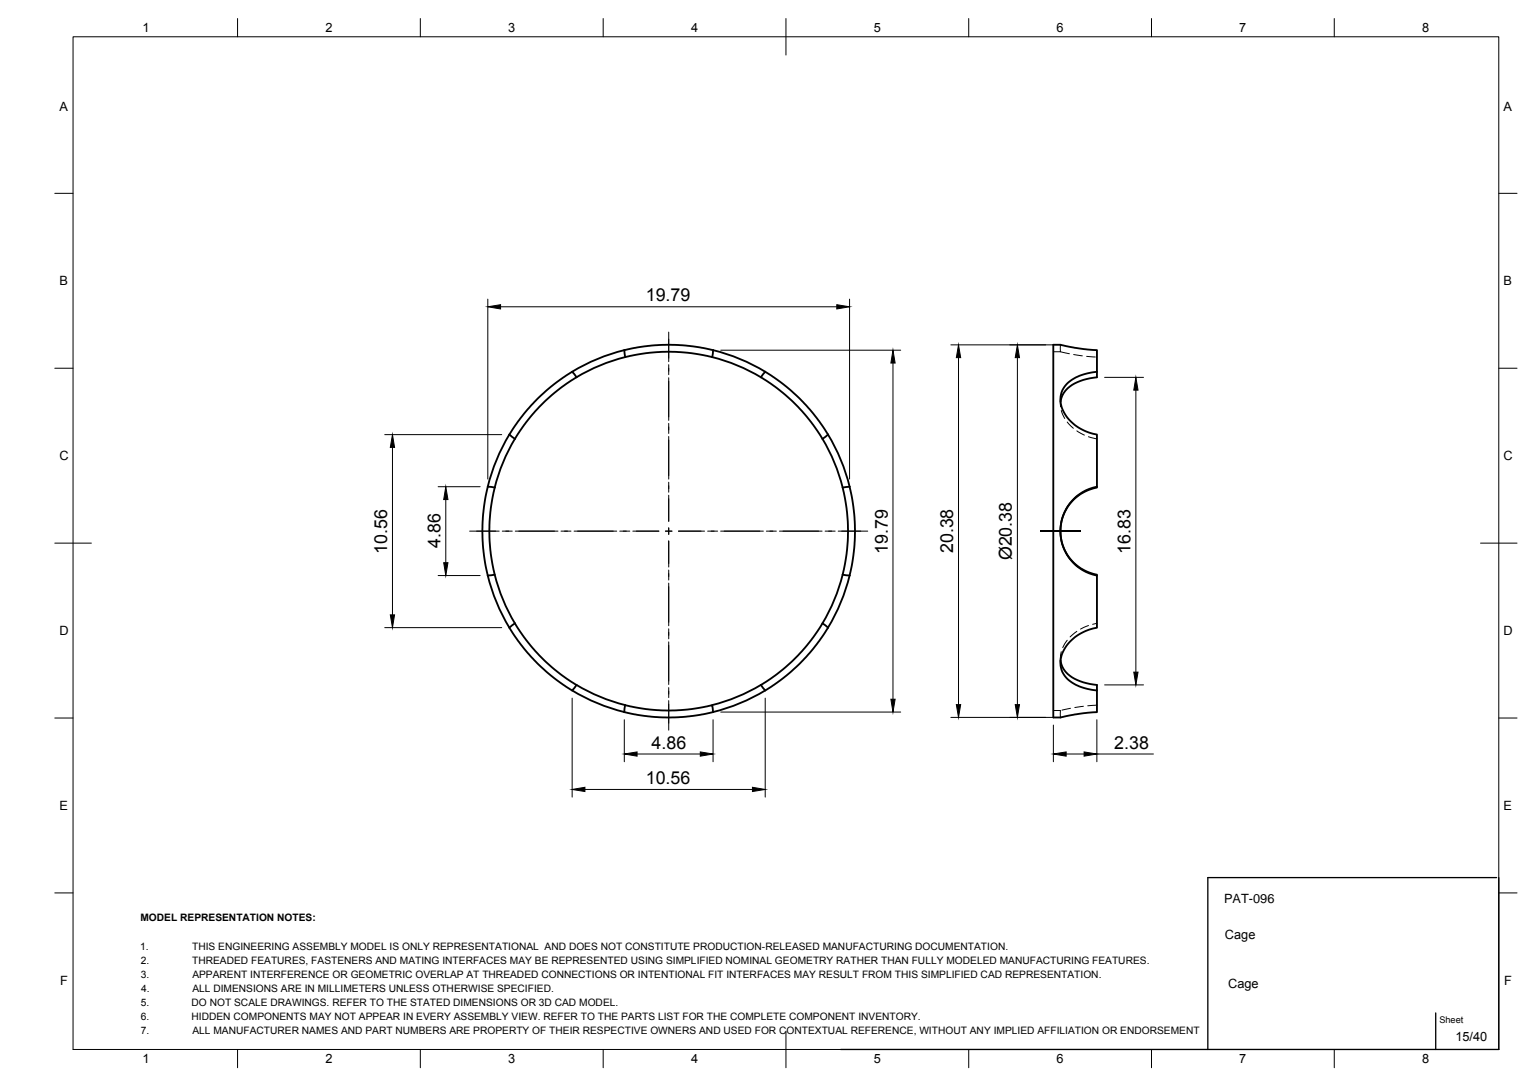
ISO-10303-21;
HEADER;
/* Generated by software containing ST-Developer
 * from STEP Tools, Inc. (www.steptools.com) 
 */

FILE_DESCRIPTION(
/* description */ ('PAT-096'),
/* implementation_level */ '2;1');

FILE_NAME(
/* name */ 'Cage.step',
/* time_stamp */ '2026-10-29T17:03:14-07:00',
/* author */ (''),
/* organization */ (''),
/* preprocessor_version */ 'ST-DEVELOPER v20.2',
/* originating_system */ 'Autodesk Translation Framework v15.17.0.0',
/* authorisation */ '');

FILE_SCHEMA (('AUTOMOTIVE_DESIGN { 1 0 10303 214 3 1 1 }'));
ENDSEC;

DATA;
#10=MECHANICAL_DESIGN_GEOMETRIC_PRESENTATION_REPRESENTATION('',(#412),#10650);
#271=SPHERICAL_SURFACE('',#6142,0.247676);
#272=SPHERICAL_SURFACE('',#6158,0.247676);
#273=SPHERICAL_SURFACE('',#6163,0.247676);
#274=SPHERICAL_SURFACE('',#6168,0.247676);
#275=SPHERICAL_SURFACE('',#6173,0.247676);
#276=SPHERICAL_SURFACE('',#6178,0.247676);
#277=SPHERICAL_SURFACE('',#6183,0.247676);
#278=SPHERICAL_SURFACE('',#6191,0.247676);
#285=B_SPLINE_CURVE_WITH_KNOTS('',3,(#9044,#9045,#9046,#9047,#9048,#9049,
#9050,#9051,#9052,#9053,#9054,#9055,#9056,#9057,#9058,#9059,#9060,#9061,
#9062,#9063,#9064,#9065),.UNSPECIFIED.,.F.,.F.,(4,2,2,2,2,2,2,2,2,2,4),
(0.0473477652366656,0.126350602536658,0.189525903804987,0.252701205073317,
0.313298422430275,0.373895639787233,0.434492857144191,0.495090074501149,
0.558265375769478,0.621440677037807,0.7004435143378),.UNSPECIFIED.);
#286=B_SPLINE_CURVE_WITH_KNOTS('',3,(#9069,#9070,#9071,#9072,#9073,#9074,
#9075,#9076,#9077,#9078,#9079,#9080,#9081,#9082,#9083,#9084,#9085,#9086,
#9087,#9088,#9089,#9090),.UNSPECIFIED.,.F.,.F.,(4,2,2,2,2,2,2,2,2,2,4),
(0.0464897534940957,0.0852567806515119,0.170513561303024,0.246687263103517,
0.308657850341199,0.370628437578881,0.432599024816563,0.494569612054245,
0.570743313854739,0.656000094506251,0.694767121663666),.UNSPECIFIED.);
#287=B_SPLINE_CURVE_WITH_KNOTS('',3,(#9096,#9097,#9098,#9099,#9100,#9101,
#9102,#9103,#9104,#9105,#9106,#9107,#9108,#9109,#9110,#9111,#9112,#9113,
#9114,#9115,#9116,#9117),.UNSPECIFIED.,.F.,.F.,(4,2,2,2,2,2,2,2,2,2,4),
(0.0464897534940957,0.0852567806515118,0.170513561303024,0.246687263103517,
0.308657850341199,0.370628437578881,0.432599024816563,0.494569612054245,
0.570743313854738,0.65600009450625,0.694767121663666),.UNSPECIFIED.);
#288=B_SPLINE_CURVE_WITH_KNOTS('',3,(#9121,#9122,#9123,#9124,#9125,#9126,
#9127,#9128,#9129,#9130,#9131,#9132,#9133,#9134,#9135,#9136,#9137,#9138,
#9139,#9140,#9141,#9142),.UNSPECIFIED.,.F.,.F.,(4,2,2,2,2,2,2,2,2,2,4),
(0.0464897534940957,0.0852567806515119,0.170513561303024,0.246687263103517,
0.308657850341199,0.370628437578881,0.432599024816563,0.494569612054245,
0.570743313854739,0.656000094506251,0.694767121663666),.UNSPECIFIED.);
#289=B_SPLINE_CURVE_WITH_KNOTS('',3,(#9146,#9147,#9148,#9149,#9150,#9151,
#9152,#9153,#9154,#9155,#9156,#9157),.UNSPECIFIED.,.F.,.F.,(4,2,2,2,2,4),
(0.0464897534940957,0.0852567806515119,0.170513561303024,0.246687263103517,
0.308657850341199,0.370628437578881),.UNSPECIFIED.);
#290=B_SPLINE_CURVE_WITH_KNOTS('',3,(#9162,#9163,#9164,#9165,#9166,#9167,
#9168,#9169,#9170,#9171,#9172,#9173),.UNSPECIFIED.,.F.,.F.,(4,2,2,2,2,4),
(0.370628437578881,0.432599024816563,0.494569612054245,0.570743313854738,
0.65600009450625,0.694767121663666),.UNSPECIFIED.);
#291=B_SPLINE_CURVE_WITH_KNOTS('',3,(#9177,#9178,#9179,#9180,#9181,#9182,
#9183,#9184,#9185,#9186,#9187,#9188,#9189,#9190,#9191,#9192,#9193,#9194,
#9195,#9196,#9197,#9198),.UNSPECIFIED.,.F.,.F.,(4,2,2,2,2,2,2,2,2,2,4),
(0.0464897534940957,0.0852567806515121,0.170513561303024,0.246687263103518,
0.308657850341199,0.370628437578881,0.432599024816563,0.494569612054245,
0.570743313854738,0.65600009450625,0.694767121663666),.UNSPECIFIED.);
#292=B_SPLINE_CURVE_WITH_KNOTS('',3,(#9202,#9203,#9204,#9205,#9206,#9207,
#9208,#9209,#9210,#9211,#9212,#9213,#9214,#9215,#9216,#9217,#9218,#9219,
#9220,#9221,#9222,#9223),.UNSPECIFIED.,.F.,.F.,(4,2,2,2,2,2,2,2,2,2,4),
(0.0464897534940957,0.0852567806515119,0.170513561303024,0.246687263103517,
0.308657850341199,0.370628437578881,0.432599024816563,0.494569612054245,
0.570743313854738,0.65600009450625,0.694767121663667),.UNSPECIFIED.);
#293=B_SPLINE_CURVE_WITH_KNOTS('',3,(#9227,#9228,#9229,#9230,#9231,#9232,
#9233,#9234,#9235,#9236,#9237,#9238,#9239,#9240,#9241,#9242,#9243,#9244,
#9245,#9246,#9247,#9248),.UNSPECIFIED.,.F.,.F.,(4,2,2,2,2,2,2,2,2,2,4),
(0.0464897534940957,0.0852567806515119,0.170513561303024,0.246687263103517,
0.308657850341199,0.370628437578881,0.432599024816563,0.494569612054245,
0.570743313854738,0.65600009450625,0.694767121663666),.UNSPECIFIED.);
#294=B_SPLINE_CURVE_WITH_KNOTS('',3,(#9252,#9253,#9254,#9255,#9256,#9257,
#9258,#9259,#9260,#9261,#9262,#9263,#9264,#9265,#9266,#9267,#9268,#9269,
#9270,#9271,#9272,#9273),.UNSPECIFIED.,.F.,.F.,(4,2,2,2,2,2,2,2,2,2,4),
(0.0464897534940957,0.0852567806515119,0.170513561303024,0.246687263103517,
0.308657850341199,0.370628437578881,0.432599024816563,0.494569612054245,
0.570743313854739,0.656000094506251,0.694767121663667),.UNSPECIFIED.);
#295=B_SPLINE_CURVE_WITH_KNOTS('',3,(#9281,#9282,#9283,#9284,#9285,#9286,
#9287,#9288,#9289,#9290,#9291,#9292,#9293,#9294,#9295,#9296,#9297,#9298,
#9299,#9300,#9301,#9302),.UNSPECIFIED.,.F.,.F.,(4,2,2,2,2,2,2,2,2,2,4),
(0.0473477652366656,0.126350602536658,0.189525903804987,0.252701205073316,
0.313298422430274,0.373895639787232,0.434492857144191,0.495090074501149,
0.558265375769478,0.621440677037807,0.7004435143378),.UNSPECIFIED.);
#296=B_SPLINE_CURVE_WITH_KNOTS('',3,(#9310,#9311,#9312,#9313,#9314,#9315,
#9316,#9317,#9318,#9319,#9320,#9321,#9322,#9323,#9324,#9325,#9326,#9327,
#9328,#9329,#9330,#9331),.UNSPECIFIED.,.F.,.F.,(4,2,2,2,2,2,2,2,2,2,4),
(0.0473477652366656,0.126350602536658,0.189525903804987,0.252701205073317,
0.313298422430275,0.373895639787233,0.434492857144191,0.495090074501149,
0.558265375769478,0.621440677037807,0.7004435143378),.UNSPECIFIED.);
#297=B_SPLINE_CURVE_WITH_KNOTS('',3,(#9340,#9341,#9342,#9343,#9344,#9345,
#9346,#9347,#9348,#9349,#9350,#9351),.UNSPECIFIED.,.F.,.F.,(4,2,2,2,2,4),
(0.0473477652366656,0.126350602536658,0.189525903804987,0.252701205073316,
0.313298422430275,0.373895639787233),.UNSPECIFIED.);
#298=B_SPLINE_CURVE_WITH_KNOTS('',3,(#9353,#9354,#9355,#9356,#9357,#9358,
#9359,#9360,#9361,#9362,#9363,#9364),.UNSPECIFIED.,.F.,.F.,(4,2,2,2,2,4),
(0.373895639787233,0.434492857144191,0.495090074501149,0.558265375769478,
0.621440677037807,0.7004435143378),.UNSPECIFIED.);
#299=B_SPLINE_CURVE_WITH_KNOTS('',3,(#9371,#9372,#9373,#9374,#9375,#9376,
#9377,#9378,#9379,#9380,#9381,#9382,#9383,#9384,#9385,#9386,#9387,#9388,
#9389,#9390,#9391,#9392),.UNSPECIFIED.,.F.,.F.,(4,2,2,2,2,2,2,2,2,2,4),
(0.0473477652366656,0.126350602536658,0.189525903804987,0.252701205073316,
0.313298422430275,0.373895639787233,0.434492857144191,0.495090074501149,
0.558265375769478,0.621440677037807,0.7004435143378),.UNSPECIFIED.);
#300=B_SPLINE_CURVE_WITH_KNOTS('',3,(#9400,#9401,#9402,#9403,#9404,#9405,
#9406,#9407,#9408,#9409,#9410,#9411,#9412,#9413,#9414,#9415,#9416,#9417,
#9418,#9419,#9420,#9421),.UNSPECIFIED.,.F.,.F.,(4,2,2,2,2,2,2,2,2,2,4),
(0.0473477652366656,0.126350602536658,0.189525903804987,0.252701205073317,
0.313298422430275,0.373895639787233,0.434492857144191,0.495090074501149,
0.558265375769478,0.621440677037807,0.7004435143378),.UNSPECIFIED.);
#301=B_SPLINE_CURVE_WITH_KNOTS('',3,(#9429,#9430,#9431,#9432,#9433,#9434,
#9435,#9436,#9437,#9438,#9439,#9440,#9441,#9442,#9443,#9444,#9445,#9446,
#9447,#9448,#9449,#9450),.UNSPECIFIED.,.F.,.F.,(4,2,2,2,2,2,2,2,2,2,4),
(0.0473477652366656,0.126350602536658,0.189525903804987,0.252701205073316,
0.313298422430275,0.373895639787233,0.434492857144191,0.495090074501149,
0.558265375769478,0.621440677037807,0.7004435143378),.UNSPECIFIED.);
#302=B_SPLINE_CURVE_WITH_KNOTS('',3,(#9459,#9460,#9461,#9462,#9463,#9464,
#9465,#9466,#9467,#9468,#9469,#9470,#9471,#9472,#9473,#9474,#9475,#9476,
#9477,#9478,#9479,#9480),.UNSPECIFIED.,.F.,.F.,(4,2,2,2,2,2,2,2,2,2,4),
(0.0473477652366656,0.126350602536658,0.189525903804987,0.252701205073317,
0.313298422430275,0.373895639787233,0.434492857144191,0.495090074501149,
0.558265375769478,0.621440677037807,0.7004435143378),.UNSPECIFIED.);
#343=SHAPE_REPRESENTATION_RELATIONSHIP('SRR','None',#10804,#374);
#374=ADVANCED_BREP_SHAPE_REPRESENTATION('',(#450),#10622);
#412=STYLED_ITEM('',(#11064),#450);
#450=MANIFOLD_SOLID_BREP('Continuous crown cage',#5546);
#527=FACE_BOUND('',#1299,.T.);
#652=PLANE('',#6155);
#653=PLANE('',#6160);
#654=PLANE('',#6165);
#655=PLANE('',#6170);
#656=PLANE('',#6175);
#657=PLANE('',#6180);
#658=PLANE('',#6189);
#659=PLANE('',#6193);
#660=PLANE('',#6194);
#891=FACE_OUTER_BOUND('',#1281,.T.);
#892=FACE_OUTER_BOUND('',#1282,.T.);
#893=FACE_OUTER_BOUND('',#1283,.T.);
#894=FACE_OUTER_BOUND('',#1284,.T.);
#895=FACE_OUTER_BOUND('',#1285,.T.);
#896=FACE_OUTER_BOUND('',#1286,.T.);
#897=FACE_OUTER_BOUND('',#1287,.T.);
#898=FACE_OUTER_BOUND('',#1288,.T.);
#899=FACE_OUTER_BOUND('',#1289,.T.);
#900=FACE_OUTER_BOUND('',#1290,.T.);
#901=FACE_OUTER_BOUND('',#1291,.T.);
#902=FACE_OUTER_BOUND('',#1292,.T.);
#903=FACE_OUTER_BOUND('',#1293,.T.);
#904=FACE_OUTER_BOUND('',#1294,.T.);
#905=FACE_OUTER_BOUND('',#1295,.T.);
#906=FACE_OUTER_BOUND('',#1296,.T.);
#907=FACE_OUTER_BOUND('',#1297,.T.);
#908=FACE_OUTER_BOUND('',#1298,.T.);
#909=FACE_OUTER_BOUND('',#1300,.T.);
#1281=EDGE_LOOP('',(#4123,#4124,#4125,#4126));
#1282=EDGE_LOOP('',(#4127,#4128,#4129,#4130,#4131,#4132,#4133,#4134,#4135,
#4136,#4137,#4138,#4139,#4140,#4141,#4142,#4143,#4144,#4145,#4146));
#1283=EDGE_LOOP('',(#4147,#4148,#4149,#4150));
#1284=EDGE_LOOP('',(#4151,#4152,#4153,#4154));
#1285=EDGE_LOOP('',(#4155,#4156,#4157,#4158));
#1286=EDGE_LOOP('',(#4159,#4160,#4161,#4162));
#1287=EDGE_LOOP('',(#4163,#4164,#4165,#4166));
#1288=EDGE_LOOP('',(#4167,#4168,#4169,#4170,#4171,#4172));
#1289=EDGE_LOOP('',(#4173,#4174,#4175,#4176));
#1290=EDGE_LOOP('',(#4177,#4178,#4179,#4180));
#1291=EDGE_LOOP('',(#4181,#4182,#4183,#4184));
#1292=EDGE_LOOP('',(#4185,#4186,#4187,#4188));
#1293=EDGE_LOOP('',(#4189,#4190,#4191,#4192));
#1294=EDGE_LOOP('',(#4193,#4194,#4195,#4196));
#1295=EDGE_LOOP('',(#4197,#4198,#4199,#4200,#4201,#4202,#4203,#4204,#4205,
#4206,#4207,#4208,#4209,#4210,#4211,#4212,#4213,#4214,#4215,#4216));
#1296=EDGE_LOOP('',(#4217,#4218,#4219,#4220));
#1297=EDGE_LOOP('',(#4221,#4222,#4223,#4224));
#1298=EDGE_LOOP('',(#4225));
#1299=EDGE_LOOP('',(#4226));
#1300=EDGE_LOOP('',(#4227,#4228,#4229,#4230));
#1686=LINE('',#9159,#2015);
#1687=LINE('',#9455,#2016);
#2015=VECTOR('',#7224,1.019052);
#2016=VECTOR('',#7301,0.980948);
#2374=CIRCLE('',#6143,0.243053047864041);
#2375=CIRCLE('',#6144,0.243053047864041);
#2376=CIRCLE('',#6146,1.019052);
#2377=CIRCLE('',#6147,1.019052);
#2378=CIRCLE('',#6148,1.019052);
#2379=CIRCLE('',#6149,1.019052);
#2380=CIRCLE('',#6150,1.019052);
#2381=CIRCLE('',#6151,1.019052);
#2382=CIRCLE('',#6152,1.019052);
#2383=CIRCLE('',#6153,1.019052);
#2384=CIRCLE('',#6154,1.019052);
#2385=CIRCLE('',#6156,0.980948);
#2386=CIRCLE('',#6157,0.243053047864041);
#2387=CIRCLE('',#6159,0.243053047864041);
#2388=CIRCLE('',#6161,0.980948);
#2389=CIRCLE('',#6162,0.243053047864041);
#2390=CIRCLE('',#6164,0.243053047864041);
#2391=CIRCLE('',#6166,0.980948);
#2392=CIRCLE('',#6167,0.243053047864041);
#2393=CIRCLE('',#6169,0.243053047864041);
#2394=CIRCLE('',#6171,0.980948);
#2395=CIRCLE('',#6172,0.243053047864041);
#2396=CIRCLE('',#6174,0.243053047864041);
#2397=CIRCLE('',#6176,0.980948);
#2398=CIRCLE('',#6177,0.243053047864041);
#2399=CIRCLE('',#6179,0.243053047864041);
#2400=CIRCLE('',#6181,0.980948);
#2401=CIRCLE('',#6182,0.243053047864041);
#2402=CIRCLE('',#6184,0.243053047864041);
#2403=CIRCLE('',#6186,0.980948);
#2404=CIRCLE('',#6187,0.980948);
#2405=CIRCLE('',#6188,0.980948);
#2406=CIRCLE('',#6190,0.243053047864041);
#2407=CIRCLE('',#6192,0.243053047864041);
#2723=VERTEX_POINT('',#9042);
#2724=VERTEX_POINT('',#9043);
#2725=VERTEX_POINT('',#9066);
#2726=VERTEX_POINT('',#9068);
#2727=VERTEX_POINT('',#9093);
#2728=VERTEX_POINT('',#9095);
#2729=VERTEX_POINT('',#9118);
#2730=VERTEX_POINT('',#9120);
#2731=VERTEX_POINT('',#9143);
#2732=VERTEX_POINT('',#9145);
#2733=VERTEX_POINT('',#9158);
#2734=VERTEX_POINT('',#9161);
#2735=VERTEX_POINT('',#9174);
#2736=VERTEX_POINT('',#9176);
#2737=VERTEX_POINT('',#9199);
#2738=VERTEX_POINT('',#9201);
#2739=VERTEX_POINT('',#9224);
#2740=VERTEX_POINT('',#9226);
#2741=VERTEX_POINT('',#9249);
#2742=VERTEX_POINT('',#9251);
#2743=VERTEX_POINT('',#9276);
#2744=VERTEX_POINT('',#9280);
#2745=VERTEX_POINT('',#9305);
#2746=VERTEX_POINT('',#9309);
#2747=VERTEX_POINT('',#9334);
#2748=VERTEX_POINT('',#9338);
#2749=VERTEX_POINT('',#9339);
#2750=VERTEX_POINT('',#9366);
#2751=VERTEX_POINT('',#9370);
#2752=VERTEX_POINT('',#9395);
#2753=VERTEX_POINT('',#9399);
#2754=VERTEX_POINT('',#9424);
#2755=VERTEX_POINT('',#9428);
#2756=VERTEX_POINT('',#9453);
#2757=VERTEX_POINT('',#9456);
#2758=VERTEX_POINT('',#9458);
#3240=EDGE_CURVE('',#2723,#2724,#285,.T.);
#3241=EDGE_CURVE('',#2725,#2723,#2374,.T.);
#3242=EDGE_CURVE('',#2726,#2725,#286,.T.);
#3243=EDGE_CURVE('',#2724,#2726,#2375,.T.);
#3244=EDGE_CURVE('',#2727,#2725,#2376,.T.);
#3245=EDGE_CURVE('',#2727,#2728,#287,.T.);
#3246=EDGE_CURVE('',#2729,#2728,#2377,.T.);
#3247=EDGE_CURVE('',#2729,#2730,#288,.T.);
#3248=EDGE_CURVE('',#2731,#2730,#2378,.T.);
#3249=EDGE_CURVE('',#2731,#2732,#289,.T.);
#3250=EDGE_CURVE('',#2732,#2733,#1686,.T.);
#3251=EDGE_CURVE('',#2733,#2733,#2379,.T.);
#3252=EDGE_CURVE('',#2732,#2734,#290,.T.);
#3253=EDGE_CURVE('',#2735,#2734,#2380,.T.);
#3254=EDGE_CURVE('',#2735,#2736,#291,.T.);
#3255=EDGE_CURVE('',#2737,#2736,#2381,.T.);
#3256=EDGE_CURVE('',#2737,#2738,#292,.T.);
#3257=EDGE_CURVE('',#2739,#2738,#2382,.T.);
#3258=EDGE_CURVE('',#2739,#2740,#293,.T.);
#3259=EDGE_CURVE('',#2741,#2740,#2383,.T.);
#3260=EDGE_CURVE('',#2741,#2742,#294,.T.);
#3261=EDGE_CURVE('',#2726,#2742,#2384,.T.);
#3262=EDGE_CURVE('',#2723,#2743,#2385,.T.);
#3263=EDGE_CURVE('',#2743,#2727,#2386,.T.);
#3264=EDGE_CURVE('',#2744,#2743,#295,.T.);
#3265=EDGE_CURVE('',#2728,#2744,#2387,.T.);
#3266=EDGE_CURVE('',#2744,#2745,#2388,.T.);
#3267=EDGE_CURVE('',#2745,#2729,#2389,.T.);
#3268=EDGE_CURVE('',#2746,#2745,#296,.T.);
#3269=EDGE_CURVE('',#2730,#2746,#2390,.T.);
#3270=EDGE_CURVE('',#2746,#2747,#2391,.T.);
#3271=EDGE_CURVE('',#2747,#2731,#2392,.T.);
#3272=EDGE_CURVE('',#2748,#2749,#297,.T.);
#3273=EDGE_CURVE('',#2734,#2748,#2393,.T.);
#3274=EDGE_CURVE('',#2749,#2747,#298,.T.);
#3275=EDGE_CURVE('',#2748,#2750,#2394,.T.);
#3276=EDGE_CURVE('',#2750,#2735,#2395,.T.);
#3277=EDGE_CURVE('',#2751,#2750,#299,.T.);
#3278=EDGE_CURVE('',#2736,#2751,#2396,.T.);
#3279=EDGE_CURVE('',#2751,#2752,#2397,.T.);
#3280=EDGE_CURVE('',#2752,#2737,#2398,.T.);
#3281=EDGE_CURVE('',#2753,#2752,#300,.T.);
#3282=EDGE_CURVE('',#2738,#2753,#2399,.T.);
#3283=EDGE_CURVE('',#2753,#2754,#2400,.T.);
#3284=EDGE_CURVE('',#2754,#2739,#2401,.T.);
#3285=EDGE_CURVE('',#2755,#2754,#301,.T.);
#3286=EDGE_CURVE('',#2740,#2755,#2402,.T.);
#3287=EDGE_CURVE('',#2756,#2756,#2403,.T.);
#3288=EDGE_CURVE('',#2756,#2749,#1687,.T.);
#3289=EDGE_CURVE('',#2757,#2724,#2404,.T.);
#3290=EDGE_CURVE('',#2757,#2758,#302,.T.);
#3291=EDGE_CURVE('',#2755,#2758,#2405,.T.);
#3292=EDGE_CURVE('',#2742,#2757,#2406,.T.);
#3293=EDGE_CURVE('',#2758,#2741,#2407,.T.);
#4123=ORIENTED_EDGE('',*,*,#3240,.F.);
#4124=ORIENTED_EDGE('',*,*,#3241,.F.);
#4125=ORIENTED_EDGE('',*,*,#3242,.F.);
#4126=ORIENTED_EDGE('',*,*,#3243,.F.);
#4127=ORIENTED_EDGE('',*,*,#3242,.T.);
#4128=ORIENTED_EDGE('',*,*,#3244,.F.);
#4129=ORIENTED_EDGE('',*,*,#3245,.T.);
#4130=ORIENTED_EDGE('',*,*,#3246,.F.);
#4131=ORIENTED_EDGE('',*,*,#3247,.T.);
#4132=ORIENTED_EDGE('',*,*,#3248,.F.);
#4133=ORIENTED_EDGE('',*,*,#3249,.T.);
#4134=ORIENTED_EDGE('',*,*,#3250,.T.);
#4135=ORIENTED_EDGE('',*,*,#3251,.F.);
#4136=ORIENTED_EDGE('',*,*,#3250,.F.);
#4137=ORIENTED_EDGE('',*,*,#3252,.T.);
#4138=ORIENTED_EDGE('',*,*,#3253,.F.);
#4139=ORIENTED_EDGE('',*,*,#3254,.T.);
#4140=ORIENTED_EDGE('',*,*,#3255,.F.);
#4141=ORIENTED_EDGE('',*,*,#3256,.T.);
#4142=ORIENTED_EDGE('',*,*,#3257,.F.);
#4143=ORIENTED_EDGE('',*,*,#3258,.T.);
#4144=ORIENTED_EDGE('',*,*,#3259,.F.);
#4145=ORIENTED_EDGE('',*,*,#3260,.T.);
#4146=ORIENTED_EDGE('',*,*,#3261,.F.);
#4147=ORIENTED_EDGE('',*,*,#3241,.T.);
#4148=ORIENTED_EDGE('',*,*,#3262,.T.);
#4149=ORIENTED_EDGE('',*,*,#3263,.T.);
#4150=ORIENTED_EDGE('',*,*,#3244,.T.);
#4151=ORIENTED_EDGE('',*,*,#3264,.F.);
#4152=ORIENTED_EDGE('',*,*,#3265,.F.);
#4153=ORIENTED_EDGE('',*,*,#3245,.F.);
#4154=ORIENTED_EDGE('',*,*,#3263,.F.);
#4155=ORIENTED_EDGE('',*,*,#3265,.T.);
#4156=ORIENTED_EDGE('',*,*,#3266,.T.);
#4157=ORIENTED_EDGE('',*,*,#3267,.T.);
#4158=ORIENTED_EDGE('',*,*,#3246,.T.);
#4159=ORIENTED_EDGE('',*,*,#3268,.F.);
#4160=ORIENTED_EDGE('',*,*,#3269,.F.);
#4161=ORIENTED_EDGE('',*,*,#3247,.F.);
#4162=ORIENTED_EDGE('',*,*,#3267,.F.);
#4163=ORIENTED_EDGE('',*,*,#3269,.T.);
#4164=ORIENTED_EDGE('',*,*,#3270,.T.);
#4165=ORIENTED_EDGE('',*,*,#3271,.T.);
#4166=ORIENTED_EDGE('',*,*,#3248,.T.);
#4167=ORIENTED_EDGE('',*,*,#3272,.F.);
#4168=ORIENTED_EDGE('',*,*,#3273,.F.);
#4169=ORIENTED_EDGE('',*,*,#3252,.F.);
#4170=ORIENTED_EDGE('',*,*,#3249,.F.);
#4171=ORIENTED_EDGE('',*,*,#3271,.F.);
#4172=ORIENTED_EDGE('',*,*,#3274,.F.);
#4173=ORIENTED_EDGE('',*,*,#3273,.T.);
#4174=ORIENTED_EDGE('',*,*,#3275,.T.);
#4175=ORIENTED_EDGE('',*,*,#3276,.T.);
#4176=ORIENTED_EDGE('',*,*,#3253,.T.);
#4177=ORIENTED_EDGE('',*,*,#3277,.F.);
#4178=ORIENTED_EDGE('',*,*,#3278,.F.);
#4179=ORIENTED_EDGE('',*,*,#3254,.F.);
#4180=ORIENTED_EDGE('',*,*,#3276,.F.);
#4181=ORIENTED_EDGE('',*,*,#3278,.T.);
#4182=ORIENTED_EDGE('',*,*,#3279,.T.);
#4183=ORIENTED_EDGE('',*,*,#3280,.T.);
#4184=ORIENTED_EDGE('',*,*,#3255,.T.);
#4185=ORIENTED_EDGE('',*,*,#3281,.F.);
#4186=ORIENTED_EDGE('',*,*,#3282,.F.);
#4187=ORIENTED_EDGE('',*,*,#3256,.F.);
#4188=ORIENTED_EDGE('',*,*,#3280,.F.);
#4189=ORIENTED_EDGE('',*,*,#3282,.T.);
#4190=ORIENTED_EDGE('',*,*,#3283,.T.);
#4191=ORIENTED_EDGE('',*,*,#3284,.T.);
#4192=ORIENTED_EDGE('',*,*,#3257,.T.);
#4193=ORIENTED_EDGE('',*,*,#3258,.F.);
#4194=ORIENTED_EDGE('',*,*,#3284,.F.);
#4195=ORIENTED_EDGE('',*,*,#3285,.F.);
#4196=ORIENTED_EDGE('',*,*,#3286,.F.);
#4197=ORIENTED_EDGE('',*,*,#3287,.F.);
#4198=ORIENTED_EDGE('',*,*,#3288,.T.);
#4199=ORIENTED_EDGE('',*,*,#3274,.T.);
#4200=ORIENTED_EDGE('',*,*,#3270,.F.);
#4201=ORIENTED_EDGE('',*,*,#3268,.T.);
#4202=ORIENTED_EDGE('',*,*,#3266,.F.);
#4203=ORIENTED_EDGE('',*,*,#3264,.T.);
#4204=ORIENTED_EDGE('',*,*,#3262,.F.);
#4205=ORIENTED_EDGE('',*,*,#3240,.T.);
#4206=ORIENTED_EDGE('',*,*,#3289,.F.);
#4207=ORIENTED_EDGE('',*,*,#3290,.T.);
#4208=ORIENTED_EDGE('',*,*,#3291,.F.);
#4209=ORIENTED_EDGE('',*,*,#3285,.T.);
#4210=ORIENTED_EDGE('',*,*,#3283,.F.);
#4211=ORIENTED_EDGE('',*,*,#3281,.T.);
#4212=ORIENTED_EDGE('',*,*,#3279,.F.);
#4213=ORIENTED_EDGE('',*,*,#3277,.T.);
#4214=ORIENTED_EDGE('',*,*,#3275,.F.);
#4215=ORIENTED_EDGE('',*,*,#3272,.T.);
#4216=ORIENTED_EDGE('',*,*,#3288,.F.);
#4217=ORIENTED_EDGE('',*,*,#3243,.T.);
#4218=ORIENTED_EDGE('',*,*,#3261,.T.);
#4219=ORIENTED_EDGE('',*,*,#3292,.T.);
#4220=ORIENTED_EDGE('',*,*,#3289,.T.);
#4221=ORIENTED_EDGE('',*,*,#3260,.F.);
#4222=ORIENTED_EDGE('',*,*,#3293,.F.);
#4223=ORIENTED_EDGE('',*,*,#3290,.F.);
#4224=ORIENTED_EDGE('',*,*,#3292,.F.);
#4225=ORIENTED_EDGE('',*,*,#3251,.T.);
#4226=ORIENTED_EDGE('',*,*,#3287,.T.);
#4227=ORIENTED_EDGE('',*,*,#3286,.T.);
#4228=ORIENTED_EDGE('',*,*,#3291,.T.);
#4229=ORIENTED_EDGE('',*,*,#3293,.T.);
#4230=ORIENTED_EDGE('',*,*,#3259,.T.);
#5117=CYLINDRICAL_SURFACE('',#6145,1.019052);
#5118=CYLINDRICAL_SURFACE('',#6185,0.980948);
#5296=ADVANCED_FACE('',(#891),#271,.F.);
#5297=ADVANCED_FACE('',(#892),#5117,.T.);
#5298=ADVANCED_FACE('',(#893),#652,.T.);
#5299=ADVANCED_FACE('',(#894),#272,.F.);
#5300=ADVANCED_FACE('',(#895),#653,.T.);
#5301=ADVANCED_FACE('',(#896),#273,.F.);
#5302=ADVANCED_FACE('',(#897),#654,.T.);
#5303=ADVANCED_FACE('',(#898),#274,.F.);
#5304=ADVANCED_FACE('',(#899),#655,.T.);
#5305=ADVANCED_FACE('',(#900),#275,.F.);
#5306=ADVANCED_FACE('',(#901),#656,.T.);
#5307=ADVANCED_FACE('',(#902),#276,.F.);
#5308=ADVANCED_FACE('',(#903),#657,.T.);
#5309=ADVANCED_FACE('',(#904),#277,.F.);
#5310=ADVANCED_FACE('',(#905),#5118,.F.);
#5311=ADVANCED_FACE('',(#906),#658,.T.);
#5312=ADVANCED_FACE('',(#907),#278,.F.);
#5313=ADVANCED_FACE('',(#908,#527),#659,.T.);
#5314=ADVANCED_FACE('',(#909),#660,.T.);
#5546=CLOSED_SHELL('',(#5296,#5297,#5298,#5299,#5300,#5301,#5302,#5303,
#5304,#5305,#5306,#5307,#5308,#5309,#5310,#5311,#5312,#5313,#5314));
#6141=AXIS2_PLACEMENT_3D('',#9040,#7208,#7209);
#6142=AXIS2_PLACEMENT_3D('',#9041,#7210,#7211);
#6143=AXIS2_PLACEMENT_3D('',#9067,#7212,#7213);
#6144=AXIS2_PLACEMENT_3D('',#9091,#7214,#7215);
#6145=AXIS2_PLACEMENT_3D('',#9092,#7216,#7217);
#6146=AXIS2_PLACEMENT_3D('',#9094,#7218,#7219);
#6147=AXIS2_PLACEMENT_3D('',#9119,#7220,#7221);
#6148=AXIS2_PLACEMENT_3D('',#9144,#7222,#7223);
#6149=AXIS2_PLACEMENT_3D('',#9160,#7225,#7226);
#6150=AXIS2_PLACEMENT_3D('',#9175,#7227,#7228);
#6151=AXIS2_PLACEMENT_3D('',#9200,#7229,#7230);
#6152=AXIS2_PLACEMENT_3D('',#9225,#7231,#7232);
#6153=AXIS2_PLACEMENT_3D('',#9250,#7233,#7234);
#6154=AXIS2_PLACEMENT_3D('',#9274,#7235,#7236);
#6155=AXIS2_PLACEMENT_3D('',#9275,#7237,#7238);
#6156=AXIS2_PLACEMENT_3D('',#9277,#7239,#7240);
#6157=AXIS2_PLACEMENT_3D('',#9278,#7241,#7242);
#6158=AXIS2_PLACEMENT_3D('',#9279,#7243,#7244);
#6159=AXIS2_PLACEMENT_3D('',#9303,#7245,#7246);
#6160=AXIS2_PLACEMENT_3D('',#9304,#7247,#7248);
#6161=AXIS2_PLACEMENT_3D('',#9306,#7249,#7250);
#6162=AXIS2_PLACEMENT_3D('',#9307,#7251,#7252);
#6163=AXIS2_PLACEMENT_3D('',#9308,#7253,#7254);
#6164=AXIS2_PLACEMENT_3D('',#9332,#7255,#7256);
#6165=AXIS2_PLACEMENT_3D('',#9333,#7257,#7258);
#6166=AXIS2_PLACEMENT_3D('',#9335,#7259,#7260);
#6167=AXIS2_PLACEMENT_3D('',#9336,#7261,#7262);
#6168=AXIS2_PLACEMENT_3D('',#9337,#7263,#7264);
#6169=AXIS2_PLACEMENT_3D('',#9352,#7265,#7266);
#6170=AXIS2_PLACEMENT_3D('',#9365,#7267,#7268);
#6171=AXIS2_PLACEMENT_3D('',#9367,#7269,#7270);
#6172=AXIS2_PLACEMENT_3D('',#9368,#7271,#7272);
#6173=AXIS2_PLACEMENT_3D('',#9369,#7273,#7274);
#6174=AXIS2_PLACEMENT_3D('',#9393,#7275,#7276);
#6175=AXIS2_PLACEMENT_3D('',#9394,#7277,#7278);
#6176=AXIS2_PLACEMENT_3D('',#9396,#7279,#7280);
#6177=AXIS2_PLACEMENT_3D('',#9397,#7281,#7282);
#6178=AXIS2_PLACEMENT_3D('',#9398,#7283,#7284);
#6179=AXIS2_PLACEMENT_3D('',#9422,#7285,#7286);
#6180=AXIS2_PLACEMENT_3D('',#9423,#7287,#7288);
#6181=AXIS2_PLACEMENT_3D('',#9425,#7289,#7290);
#6182=AXIS2_PLACEMENT_3D('',#9426,#7291,#7292);
#6183=AXIS2_PLACEMENT_3D('',#9427,#7293,#7294);
#6184=AXIS2_PLACEMENT_3D('',#9451,#7295,#7296);
#6185=AXIS2_PLACEMENT_3D('',#9452,#7297,#7298);
#6186=AXIS2_PLACEMENT_3D('',#9454,#7299,#7300);
#6187=AXIS2_PLACEMENT_3D('',#9457,#7302,#7303);
#6188=AXIS2_PLACEMENT_3D('',#9481,#7304,#7305);
#6189=AXIS2_PLACEMENT_3D('',#9482,#7306,#7307);
#6190=AXIS2_PLACEMENT_3D('',#9483,#7308,#7309);
#6191=AXIS2_PLACEMENT_3D('',#9484,#7310,#7311);
#6192=AXIS2_PLACEMENT_3D('',#9485,#7312,#7313);
#6193=AXIS2_PLACEMENT_3D('',#9486,#7314,#7315);
#6194=AXIS2_PLACEMENT_3D('',#9487,#7316,#7317);
#7208=DIRECTION('axis',(0.,0.,1.));
#7209=DIRECTION('refdir',(1.,0.,0.));
#7210=DIRECTION('center_axis',(0.,0.,1.));
#7211=DIRECTION('ref_axis',(1.,0.,0.));
#7212=DIRECTION('center_axis',(0.,-1.,0.));
#7213=DIRECTION('ref_axis',(0.,0.,-1.));
#7214=DIRECTION('center_axis',(0.,-1.,0.));
#7215=DIRECTION('ref_axis',(0.,0.,-1.));
#7216=DIRECTION('center_axis',(0.,1.,0.));
#7217=DIRECTION('ref_axis',(1.,0.,0.));
#7218=DIRECTION('center_axis',(0.,1.,0.));
#7219=DIRECTION('ref_axis',(1.,0.,0.));
#7220=DIRECTION('center_axis',(0.,1.,0.));
#7221=DIRECTION('ref_axis',(1.,0.,0.));
#7222=DIRECTION('center_axis',(0.,1.,0.));
#7223=DIRECTION('ref_axis',(1.,0.,0.));
#7224=DIRECTION('',(0.,-1.,0.));
#7225=DIRECTION('center_axis',(0.,-1.,0.));
#7226=DIRECTION('ref_axis',(1.,0.,0.));
#7227=DIRECTION('center_axis',(0.,1.,0.));
#7228=DIRECTION('ref_axis',(1.,0.,0.));
#7229=DIRECTION('center_axis',(0.,1.,0.));
#7230=DIRECTION('ref_axis',(1.,0.,0.));
#7231=DIRECTION('center_axis',(0.,1.,0.));
#7232=DIRECTION('ref_axis',(1.,0.,0.));
#7233=DIRECTION('center_axis',(0.,1.,0.));
#7234=DIRECTION('ref_axis',(1.,0.,0.));
#7235=DIRECTION('center_axis',(0.,1.,0.));
#7236=DIRECTION('ref_axis',(1.,0.,0.));
#7237=DIRECTION('center_axis',(0.,1.,0.));
#7238=DIRECTION('ref_axis',(1.,0.,0.));
#7239=DIRECTION('center_axis',(0.,-1.,0.));
#7240=DIRECTION('ref_axis',(1.,0.,0.));
#7241=DIRECTION('center_axis',(0.,-1.,0.));
#7242=DIRECTION('ref_axis',(0.,0.,-1.));
#7243=DIRECTION('center_axis',(6.12323399573677E-17,0.,1.));
#7244=DIRECTION('ref_axis',(1.,0.,0.));
#7245=DIRECTION('center_axis',(0.,-1.,0.));
#7246=DIRECTION('ref_axis',(0.,0.,-1.));
#7247=DIRECTION('center_axis',(0.,1.,0.));
#7248=DIRECTION('ref_axis',(1.,0.,0.));
#7249=DIRECTION('center_axis',(0.,-1.,0.));
#7250=DIRECTION('ref_axis',(1.,0.,0.));
#7251=DIRECTION('center_axis',(0.,-1.,0.));
#7252=DIRECTION('ref_axis',(0.,0.,-1.));
#7253=DIRECTION('center_axis',(0.,0.,1.));
#7254=DIRECTION('ref_axis',(1.,0.,0.));
#7255=DIRECTION('center_axis',(0.,-1.,0.));
#7256=DIRECTION('ref_axis',(0.,0.,-1.));
#7257=DIRECTION('center_axis',(0.,1.,0.));
#7258=DIRECTION('ref_axis',(1.,0.,0.));
#7259=DIRECTION('center_axis',(0.,-1.,0.));
#7260=DIRECTION('ref_axis',(1.,0.,0.));
#7261=DIRECTION('center_axis',(0.,-1.,0.));
#7262=DIRECTION('ref_axis',(0.,0.,-1.));
#7263=DIRECTION('center_axis',(0.,0.,1.));
#7264=DIRECTION('ref_axis',(1.,0.,0.));
#7265=DIRECTION('center_axis',(0.,-1.,0.));
#7266=DIRECTION('ref_axis',(0.,0.,-1.));
#7267=DIRECTION('center_axis',(0.,1.,0.));
#7268=DIRECTION('ref_axis',(1.,0.,0.));
#7269=DIRECTION('center_axis',(0.,-1.,0.));
#7270=DIRECTION('ref_axis',(1.,0.,0.));
#7271=DIRECTION('center_axis',(0.,-1.,0.));
#7272=DIRECTION('ref_axis',(0.,0.,-1.));
#7273=DIRECTION('center_axis',(0.,0.,1.));
#7274=DIRECTION('ref_axis',(1.,0.,0.));
#7275=DIRECTION('center_axis',(0.,-1.,0.));
#7276=DIRECTION('ref_axis',(0.,0.,-1.));
#7277=DIRECTION('center_axis',(0.,1.,0.));
#7278=DIRECTION('ref_axis',(1.,0.,0.));
#7279=DIRECTION('center_axis',(0.,-1.,0.));
#7280=DIRECTION('ref_axis',(1.,0.,0.));
#7281=DIRECTION('center_axis',(0.,-1.,0.));
#7282=DIRECTION('ref_axis',(0.,0.,-1.));
#7283=DIRECTION('center_axis',(6.12323399573676E-17,0.,1.));
#7284=DIRECTION('ref_axis',(1.,0.,0.));
#7285=DIRECTION('center_axis',(0.,-1.,0.));
#7286=DIRECTION('ref_axis',(0.,0.,-1.));
#7287=DIRECTION('center_axis',(0.,1.,0.));
#7288=DIRECTION('ref_axis',(1.,0.,0.));
#7289=DIRECTION('center_axis',(0.,-1.,0.));
#7290=DIRECTION('ref_axis',(1.,0.,0.));
#7291=DIRECTION('center_axis',(0.,-1.,0.));
#7292=DIRECTION('ref_axis',(0.,0.,-1.));
#7293=DIRECTION('center_axis',(0.,0.,1.));
#7294=DIRECTION('ref_axis',(1.,0.,0.));
#7295=DIRECTION('center_axis',(0.,-1.,0.));
#7296=DIRECTION('ref_axis',(0.,0.,-1.));
#7297=DIRECTION('center_axis',(0.,1.,0.));
#7298=DIRECTION('ref_axis',(1.,0.,0.));
#7299=DIRECTION('center_axis',(0.,1.,0.));
#7300=DIRECTION('ref_axis',(1.,0.,0.));
#7301=DIRECTION('',(0.,1.,0.));
#7302=DIRECTION('center_axis',(0.,-1.,0.));
#7303=DIRECTION('ref_axis',(1.,0.,0.));
#7304=DIRECTION('center_axis',(0.,-1.,0.));
#7305=DIRECTION('ref_axis',(1.,0.,0.));
#7306=DIRECTION('center_axis',(0.,1.,0.));
#7307=DIRECTION('ref_axis',(1.,0.,0.));
#7308=DIRECTION('center_axis',(0.,-1.,0.));
#7309=DIRECTION('ref_axis',(0.,0.,-1.));
#7310=DIRECTION('center_axis',(0.,0.,1.));
#7311=DIRECTION('ref_axis',(1.,0.,0.));
#7312=DIRECTION('center_axis',(0.,-1.,0.));
#7313=DIRECTION('ref_axis',(0.,0.,-1.));
#7314=DIRECTION('center_axis',(0.,-1.,0.));
#7315=DIRECTION('ref_axis',(-1.,0.,0.));
#7316=DIRECTION('center_axis',(0.,1.,0.));
#7317=DIRECTION('ref_axis',(1.,0.,0.));
#9040=CARTESIAN_POINT('',(0.,0.,0.));
#9041=CARTESIAN_POINT('Origin',(0.707106781186547,0.,0.707106781186548));
#9042=CARTESIAN_POINT('',(0.504455939115715,-0.04763,0.841298510752802));
#9043=CARTESIAN_POINT('',(0.841298510752802,-0.04763,0.504455939115715));
#9044=CARTESIAN_POINT('Ctrl Pts',(0.504455939115715,-0.04763,0.841298510752802));
#9045=CARTESIAN_POINT('Ctrl Pts',(0.508899795931835,-0.0740444353928835,
0.838633903678357));
#9046=CARTESIAN_POINT('Ctrl Pts',(0.517157748491652,-0.0999305678883309,
0.833661031856294));
#9047=CARTESIAN_POINT('Ctrl Pts',(0.537715343527944,-0.142345102874864,
0.820511285096538));
#9048=CARTESIAN_POINT('Ctrl Pts',(0.548874290046456,-0.159766064500479,
0.813159949759));
#9049=CARTESIAN_POINT('Ctrl Pts',(0.573915184558107,-0.190326085855194,
0.795684265985089));
#9050=CARTESIAN_POINT('Ctrl Pts',(0.587792702767295,-0.203463743702801,
0.78555112003688));
#9051=CARTESIAN_POINT('Ctrl Pts',(0.615966552324775,-0.224161999508995,
0.763642258217233));
#9052=CARTESIAN_POINT('Ctrl Pts',(0.631684198665438,-0.232861760990032,
0.750785745543687));
#9053=CARTESIAN_POINT('Ctrl Pts',(0.663382628119203,-0.244251601209411,
0.722929908501543));
#9054=CARTESIAN_POINT('Ctrl Pts',(0.679352081686668,-0.246942143572133,
0.707917883896095));
#9055=CARTESIAN_POINT('Ctrl Pts',(0.707917883896095,-0.246942143572133,
0.679352081686668));
#9056=CARTESIAN_POINT('Ctrl Pts',(0.722929908501543,-0.244251601209411,
0.663382628119203));
#9057=CARTESIAN_POINT('Ctrl Pts',(0.750785745543687,-0.232861760990032,
0.631684198665439));
#9058=CARTESIAN_POINT('Ctrl Pts',(0.763642258217232,-0.224161999508995,
0.615966552324775));
#9059=CARTESIAN_POINT('Ctrl Pts',(0.78555112003688,-0.203463743702801,0.587792702767295));
#9060=CARTESIAN_POINT('Ctrl Pts',(0.795684265985088,-0.190326085855194,
0.573915184558108));
#9061=CARTESIAN_POINT('Ctrl Pts',(0.813159949759,-0.15976606450048,0.548874290046456));
#9062=CARTESIAN_POINT('Ctrl Pts',(0.820511285096538,-0.142345102874864,
0.537715343527944));
#9063=CARTESIAN_POINT('Ctrl Pts',(0.833661031856294,-0.099930567888331,
0.517157748491653));
#9064=CARTESIAN_POINT('Ctrl Pts',(0.838633903678357,-0.0740444353928835,
0.508899795931835));
#9065=CARTESIAN_POINT('Ctrl Pts',(0.841298510752801,-0.0476299999999999,
0.504455939115715));
#9066=CARTESIAN_POINT('',(0.528110872004958,-0.04763,0.871530771444223));
#9067=CARTESIAN_POINT('Origin',(0.707106781186547,-0.04763,0.707106781186548));
#9068=CARTESIAN_POINT('',(0.871530771444223,-0.04763,0.528110872004959));
#9069=CARTESIAN_POINT('Ctrl Pts',(0.871530771444223,-0.0476300000000001,
0.528110872004958));
#9070=CARTESIAN_POINT('Ctrl Pts',(0.87014664509073,-0.0609922781173483,
0.530395067942936));
#9071=CARTESIAN_POINT('Ctrl Pts',(0.868149331745851,-0.0742967091364493,
0.533674141594226));
#9072=CARTESIAN_POINT('Ctrl Pts',(0.85981294420286,-0.115492077056649,0.54708917182331));
#9073=CARTESIAN_POINT('Ctrl Pts',(0.850993704737257,-0.141695629206859,
0.560922177770136));
#9074=CARTESIAN_POINT('Ctrl Pts',(0.830754510485543,-0.181890537957859,
0.590422647829571));
#9075=CARTESIAN_POINT('Ctrl Pts',(0.816896541396381,-0.201072148666545,
0.609616703125488));
#9076=CARTESIAN_POINT('Ctrl Pts',(0.792310597819928,-0.223955109275652,
0.641117951819998));
#9077=CARTESIAN_POINT('Ctrl Pts',(0.779109323683612,-0.232742381310829,
0.657208095763053));
#9078=CARTESIAN_POINT('Ctrl Pts',(0.750552691816206,-0.244234834628584,
0.68964083160521));
#9079=CARTESIAN_POINT('Ctrl Pts',(0.735185187071673,-0.246942143572133,
0.705971972091755));
#9080=CARTESIAN_POINT('Ctrl Pts',(0.705971972091754,-0.246942143572133,
0.735185187071673));
#9081=CARTESIAN_POINT('Ctrl Pts',(0.689640831605209,-0.244234834628584,
0.750552691816206));
#9082=CARTESIAN_POINT('Ctrl Pts',(0.657208095763052,-0.232742381310829,
0.779109323683612));
#9083=CARTESIAN_POINT('Ctrl Pts',(0.641117951819998,-0.223955109275652,
0.792310597819928));
#9084=CARTESIAN_POINT('Ctrl Pts',(0.609616703125487,-0.201072148666545,
0.816896541396382));
#9085=CARTESIAN_POINT('Ctrl Pts',(0.590422647829571,-0.181890537957858,
0.830754510485544));
#9086=CARTESIAN_POINT('Ctrl Pts',(0.560922177770135,-0.141695629206858,
0.850993704737257));
#9087=CARTESIAN_POINT('Ctrl Pts',(0.547089171823309,-0.115492077056649,
0.859812944202861));
#9088=CARTESIAN_POINT('Ctrl Pts',(0.533674141594226,-0.0742967091364491,
0.868149331745852));
#9089=CARTESIAN_POINT('Ctrl Pts',(0.530395067942936,-0.0609922781173483,
0.870146645090731));
#9090=CARTESIAN_POINT('Ctrl Pts',(0.528110872004958,-0.0476300000000001,
0.871530771444223));
#9091=CARTESIAN_POINT('Origin',(0.707106781186547,-0.04763,0.707106781186548));
#9092=CARTESIAN_POINT('Origin',(0.,-0.166705,0.));
#9093=CARTESIAN_POINT('',(0.242834539687906,-0.04763,0.989696097314));
#9094=CARTESIAN_POINT('Origin',(0.,-0.04763,0.));
#9095=CARTESIAN_POINT('',(-0.242834539687907,-0.04763,0.989696097314));
#9096=CARTESIAN_POINT('Ctrl Pts',(0.242834539687906,-0.04763,0.989696097314));
#9097=CARTESIAN_POINT('Ctrl Pts',(0.24024064412003,-0.0609922781173483,
0.990332542620729));
#9098=CARTESIAN_POINT('Ctrl Pts',(0.236509675094874,-0.0742967091364492,
0.991238884025248));
#9099=CARTESIAN_POINT('Ctrl Pts',(0.221129100087819,-0.115492077056649,
0.994830026707808));
#9100=CARTESIAN_POINT('Ctrl Pts',(0.205111543747588,-0.141695629206859,
0.998375294985966));
#9101=CARTESIAN_POINT('Ctrl Pts',(0.169940289819232,-0.181890537957859,
1.00492400591205));
#9102=CARTESIAN_POINT('Ctrl Pts',(0.1465689792446,-0.201072148666545,1.00869718865384));
#9103=CARTESIAN_POINT('Ctrl Pts',(0.106909345252087,-0.223955109275652,
1.01358704779679));
#9104=CARTESIAN_POINT('Ctrl Pts',(0.0861971848975941,-0.232742381310829,
1.0156297872271));
#9105=CARTESIAN_POINT('Ctrl Pts',(0.0430711894098822,-0.244234834628584,
1.01837060663223));
#9106=CARTESIAN_POINT('Ctrl Pts',(0.0206568624125605,-0.246942143572133,
1.019052));
#9107=CARTESIAN_POINT('Ctrl Pts',(-0.0206568624125608,-0.246942143572133,
1.019052));
#9108=CARTESIAN_POINT('Ctrl Pts',(-0.0430711894098825,-0.244234834628584,
1.01837060663223));
#9109=CARTESIAN_POINT('Ctrl Pts',(-0.0861971848975943,-0.232742381310829,
1.0156297872271));
#9110=CARTESIAN_POINT('Ctrl Pts',(-0.106909345252088,-0.223955109275652,
1.01358704779679));
#9111=CARTESIAN_POINT('Ctrl Pts',(-0.1465689792446,-0.201072148666545,1.00869718865384));
#9112=CARTESIAN_POINT('Ctrl Pts',(-0.169940289819232,-0.181890537957859,
1.00492400591205));
#9113=CARTESIAN_POINT('Ctrl Pts',(-0.205111543747588,-0.141695629206859,
0.998375294985966));
#9114=CARTESIAN_POINT('Ctrl Pts',(-0.221129100087819,-0.115492077056649,
0.994830026707808));
#9115=CARTESIAN_POINT('Ctrl Pts',(-0.236509675094875,-0.0742967091364493,
0.991238884025248));
#9116=CARTESIAN_POINT('Ctrl Pts',(-0.24024064412003,-0.0609922781173483,
0.990332542620729));
#9117=CARTESIAN_POINT('Ctrl Pts',(-0.242834539687907,-0.04763,0.989696097314));
#9118=CARTESIAN_POINT('',(-0.528110872004959,-0.04763,0.871530771444223));
#9119=CARTESIAN_POINT('Origin',(0.,-0.04763,0.));
#9120=CARTESIAN_POINT('',(-0.871530771444223,-0.04763,0.528110872004958));
#9121=CARTESIAN_POINT('Ctrl Pts',(-0.528110872004958,-0.0476300000000001,
0.871530771444223));
#9122=CARTESIAN_POINT('Ctrl Pts',(-0.530395067942936,-0.0609922781173484,
0.87014664509073));
#9123=CARTESIAN_POINT('Ctrl Pts',(-0.533674141594226,-0.0742967091364493,
0.868149331745851));
#9124=CARTESIAN_POINT('Ctrl Pts',(-0.54708917182331,-0.115492077056649,
0.85981294420286));
#9125=CARTESIAN_POINT('Ctrl Pts',(-0.560922177770136,-0.141695629206859,
0.850993704737257));
#9126=CARTESIAN_POINT('Ctrl Pts',(-0.590422647829571,-0.181890537957859,
0.830754510485543));
#9127=CARTESIAN_POINT('Ctrl Pts',(-0.609616703125488,-0.201072148666545,
0.816896541396381));
#9128=CARTESIAN_POINT('Ctrl Pts',(-0.641117951819998,-0.223955109275652,
0.792310597819928));
#9129=CARTESIAN_POINT('Ctrl Pts',(-0.657208095763053,-0.232742381310829,
0.779109323683611));
#9130=CARTESIAN_POINT('Ctrl Pts',(-0.68964083160521,-0.244234834628584,
0.750552691816205));
#9131=CARTESIAN_POINT('Ctrl Pts',(-0.705971972091755,-0.246942143572133,
0.735185187071673));
#9132=CARTESIAN_POINT('Ctrl Pts',(-0.735185187071673,-0.246942143572133,
0.705971972091754));
#9133=CARTESIAN_POINT('Ctrl Pts',(-0.750552691816206,-0.244234834628584,
0.689640831605209));
#9134=CARTESIAN_POINT('Ctrl Pts',(-0.779109323683612,-0.232742381310829,
0.657208095763052));
#9135=CARTESIAN_POINT('Ctrl Pts',(-0.792310597819928,-0.223955109275652,
0.641117951819998));
#9136=CARTESIAN_POINT('Ctrl Pts',(-0.816896541396382,-0.201072148666545,
0.609616703125487));
#9137=CARTESIAN_POINT('Ctrl Pts',(-0.830754510485544,-0.181890537957858,
0.590422647829571));
#9138=CARTESIAN_POINT('Ctrl Pts',(-0.850993704737257,-0.141695629206858,
0.560922177770135));
#9139=CARTESIAN_POINT('Ctrl Pts',(-0.859812944202861,-0.115492077056649,
0.547089171823309));
#9140=CARTESIAN_POINT('Ctrl Pts',(-0.868149331745852,-0.0742967091364491,
0.533674141594226));
#9141=CARTESIAN_POINT('Ctrl Pts',(-0.870146645090731,-0.0609922781173483,
0.530395067942936));
#9142=CARTESIAN_POINT('Ctrl Pts',(-0.871530771444223,-0.04763,0.528110872004958));
#9143=CARTESIAN_POINT('',(-0.989696097314,-0.04763,0.242834539687906));
#9144=CARTESIAN_POINT('Origin',(0.,-0.04763,0.));
#9145=CARTESIAN_POINT('',(-1.019052,-0.246942143572133,1.248489836334E-16));
#9146=CARTESIAN_POINT('Ctrl Pts',(-0.989696097314,-0.04763,0.242834539687906));
#9147=CARTESIAN_POINT('Ctrl Pts',(-0.990332542620729,-0.0609922781173483,
0.24024064412003));
#9148=CARTESIAN_POINT('Ctrl Pts',(-0.991238884025248,-0.0742967091364492,
0.236509675094874));
#9149=CARTESIAN_POINT('Ctrl Pts',(-0.994830026707808,-0.115492077056649,
0.221129100087819));
#9150=CARTESIAN_POINT('Ctrl Pts',(-0.998375294985966,-0.141695629206859,
0.205111543747588));
#9151=CARTESIAN_POINT('Ctrl Pts',(-1.00492400591205,-0.181890537957859,
0.169940289819232));
#9152=CARTESIAN_POINT('Ctrl Pts',(-1.00869718865384,-0.201072148666545,
0.1465689792446));
#9153=CARTESIAN_POINT('Ctrl Pts',(-1.01358704779679,-0.223955109275652,
0.106909345252088));
#9154=CARTESIAN_POINT('Ctrl Pts',(-1.0156297872271,-0.232742381310829,0.0861971848975944));
#9155=CARTESIAN_POINT('Ctrl Pts',(-1.01837060663223,-0.244234834628584,
0.0430711894098825));
#9156=CARTESIAN_POINT('Ctrl Pts',(-1.019052,-0.246942143572133,0.0206568624125608));
#9157=CARTESIAN_POINT('Ctrl Pts',(-1.019052,-0.246942143572133,1.2490009027033E-16));
#9158=CARTESIAN_POINT('',(-1.019052,-0.28578,1.24797876996471E-16));
#9159=CARTESIAN_POINT('',(-1.019052,-0.166705,1.24797876996471E-16));
#9160=CARTESIAN_POINT('Origin',(0.,-0.28578,0.));
#9161=CARTESIAN_POINT('',(-0.989696097314,-0.04763,-0.242834539687906));
#9162=CARTESIAN_POINT('Ctrl Pts',(-1.019052,-0.246942143572133,1.2490009027033E-16));
#9163=CARTESIAN_POINT('Ctrl Pts',(-1.019052,-0.246942143572133,-0.0206568624125605));
#9164=CARTESIAN_POINT('Ctrl Pts',(-1.01837060663223,-0.244234834628584,
-0.0430711894098822));
#9165=CARTESIAN_POINT('Ctrl Pts',(-1.0156297872271,-0.232742381310829,-0.0861971848975941));
#9166=CARTESIAN_POINT('Ctrl Pts',(-1.01358704779679,-0.223955109275652,
-0.106909345252087));
#9167=CARTESIAN_POINT('Ctrl Pts',(-1.00869718865384,-0.201072148666546,
-0.1465689792446));
#9168=CARTESIAN_POINT('Ctrl Pts',(-1.00492400591205,-0.181890537957859,
-0.169940289819232));
#9169=CARTESIAN_POINT('Ctrl Pts',(-0.998375294985966,-0.141695629206859,
-0.205111543747588));
#9170=CARTESIAN_POINT('Ctrl Pts',(-0.994830026707808,-0.11549207705665,
-0.221129100087819));
#9171=CARTESIAN_POINT('Ctrl Pts',(-0.991238884025248,-0.0742967091364495,
-0.236509675094874));
#9172=CARTESIAN_POINT('Ctrl Pts',(-0.990332542620729,-0.0609922781173484,
-0.24024064412003));
#9173=CARTESIAN_POINT('Ctrl Pts',(-0.989696097314,-0.0476300000000001,-0.242834539687907));
#9174=CARTESIAN_POINT('',(-0.871530771444223,-0.04763,-0.528110872004958));
#9175=CARTESIAN_POINT('Origin',(0.,-0.04763,0.));
#9176=CARTESIAN_POINT('',(-0.528110872004958,-0.04763,-0.871530771444223));
#9177=CARTESIAN_POINT('Ctrl Pts',(-0.871530771444223,-0.0476300000000001,
-0.528110872004958));
#9178=CARTESIAN_POINT('Ctrl Pts',(-0.87014664509073,-0.0609922781173484,
-0.530395067942936));
#9179=CARTESIAN_POINT('Ctrl Pts',(-0.868149331745851,-0.0742967091364494,
-0.533674141594226));
#9180=CARTESIAN_POINT('Ctrl Pts',(-0.85981294420286,-0.115492077056649,
-0.54708917182331));
#9181=CARTESIAN_POINT('Ctrl Pts',(-0.850993704737257,-0.141695629206859,
-0.560922177770136));
#9182=CARTESIAN_POINT('Ctrl Pts',(-0.830754510485543,-0.181890537957859,
-0.590422647829571));
#9183=CARTESIAN_POINT('Ctrl Pts',(-0.816896541396381,-0.201072148666546,
-0.609616703125488));
#9184=CARTESIAN_POINT('Ctrl Pts',(-0.792310597819928,-0.223955109275652,
-0.641117951819999));
#9185=CARTESIAN_POINT('Ctrl Pts',(-0.779109323683611,-0.232742381310829,
-0.657208095763053));
#9186=CARTESIAN_POINT('Ctrl Pts',(-0.750552691816205,-0.244234834628584,
-0.68964083160521));
#9187=CARTESIAN_POINT('Ctrl Pts',(-0.735185187071673,-0.246942143572133,
-0.705971972091755));
#9188=CARTESIAN_POINT('Ctrl Pts',(-0.705971972091754,-0.246942143572133,
-0.735185187071673));
#9189=CARTESIAN_POINT('Ctrl Pts',(-0.68964083160521,-0.244234834628584,
-0.750552691816206));
#9190=CARTESIAN_POINT('Ctrl Pts',(-0.657208095763052,-0.232742381310829,
-0.779109323683612));
#9191=CARTESIAN_POINT('Ctrl Pts',(-0.641117951819998,-0.223955109275652,
-0.792310597819928));
#9192=CARTESIAN_POINT('Ctrl Pts',(-0.609616703125488,-0.201072148666545,
-0.816896541396381));
#9193=CARTESIAN_POINT('Ctrl Pts',(-0.590422647829571,-0.181890537957859,
-0.830754510485543));
#9194=CARTESIAN_POINT('Ctrl Pts',(-0.560922177770136,-0.141695629206859,
-0.850993704737257));
#9195=CARTESIAN_POINT('Ctrl Pts',(-0.54708917182331,-0.115492077056649,
-0.85981294420286));
#9196=CARTESIAN_POINT('Ctrl Pts',(-0.533674141594226,-0.0742967091364494,
-0.868149331745852));
#9197=CARTESIAN_POINT('Ctrl Pts',(-0.530395067942936,-0.0609922781173484,
-0.870146645090731));
#9198=CARTESIAN_POINT('Ctrl Pts',(-0.528110872004958,-0.0476300000000001,
-0.871530771444223));
#9199=CARTESIAN_POINT('',(-0.242834539687906,-0.04763,-0.989696097314));
#9200=CARTESIAN_POINT('Origin',(0.,-0.04763,0.));
#9201=CARTESIAN_POINT('',(0.242834539687906,-0.04763,-0.989696097314));
#9202=CARTESIAN_POINT('Ctrl Pts',(-0.242834539687907,-0.04763,-0.989696097314));
#9203=CARTESIAN_POINT('Ctrl Pts',(-0.24024064412003,-0.0609922781173483,
-0.990332542620729));
#9204=CARTESIAN_POINT('Ctrl Pts',(-0.236509675094874,-0.0742967091364493,
-0.991238884025248));
#9205=CARTESIAN_POINT('Ctrl Pts',(-0.221129100087819,-0.115492077056649,
-0.994830026707808));
#9206=CARTESIAN_POINT('Ctrl Pts',(-0.205111543747588,-0.141695629206859,
-0.998375294985966));
#9207=CARTESIAN_POINT('Ctrl Pts',(-0.169940289819232,-0.181890537957859,
-1.00492400591205));
#9208=CARTESIAN_POINT('Ctrl Pts',(-0.1465689792446,-0.201072148666545,-1.00869718865384));
#9209=CARTESIAN_POINT('Ctrl Pts',(-0.106909345252087,-0.223955109275652,
-1.01358704779679));
#9210=CARTESIAN_POINT('Ctrl Pts',(-0.0861971848975942,-0.232742381310829,
-1.0156297872271));
#9211=CARTESIAN_POINT('Ctrl Pts',(-0.0430711894098823,-0.244234834628584,
-1.01837060663223));
#9212=CARTESIAN_POINT('Ctrl Pts',(-0.0206568624125606,-0.246942143572133,
-1.019052));
#9213=CARTESIAN_POINT('Ctrl Pts',(0.0206568624125607,-0.246942143572133,
-1.019052));
#9214=CARTESIAN_POINT('Ctrl Pts',(0.0430711894098824,-0.244234834628584,
-1.01837060663223));
#9215=CARTESIAN_POINT('Ctrl Pts',(0.0861971848975943,-0.232742381310829,
-1.0156297872271));
#9216=CARTESIAN_POINT('Ctrl Pts',(0.106909345252088,-0.223955109275652,
-1.01358704779679));
#9217=CARTESIAN_POINT('Ctrl Pts',(0.1465689792446,-0.201072148666545,-1.00869718865384));
#9218=CARTESIAN_POINT('Ctrl Pts',(0.169940289819232,-0.181890537957859,
-1.00492400591205));
#9219=CARTESIAN_POINT('Ctrl Pts',(0.205111543747588,-0.141695629206859,
-0.998375294985966));
#9220=CARTESIAN_POINT('Ctrl Pts',(0.221129100087819,-0.115492077056649,
-0.994830026707808));
#9221=CARTESIAN_POINT('Ctrl Pts',(0.236509675094874,-0.0742967091364493,
-0.991238884025248));
#9222=CARTESIAN_POINT('Ctrl Pts',(0.24024064412003,-0.0609922781173484,
-0.990332542620729));
#9223=CARTESIAN_POINT('Ctrl Pts',(0.242834539687907,-0.04763,-0.989696097314));
#9224=CARTESIAN_POINT('',(0.528110872004958,-0.04763,-0.871530771444223));
#9225=CARTESIAN_POINT('Origin',(0.,-0.04763,0.));
#9226=CARTESIAN_POINT('',(0.871530771444223,-0.04763,-0.528110872004958));
#9227=CARTESIAN_POINT('Ctrl Pts',(0.528110872004958,-0.0476300000000001,
-0.871530771444223));
#9228=CARTESIAN_POINT('Ctrl Pts',(0.530395067942936,-0.0609922781173484,
-0.870146645090731));
#9229=CARTESIAN_POINT('Ctrl Pts',(0.533674141594226,-0.0742967091364493,
-0.868149331745851));
#9230=CARTESIAN_POINT('Ctrl Pts',(0.54708917182331,-0.115492077056649,-0.85981294420286));
#9231=CARTESIAN_POINT('Ctrl Pts',(0.560922177770136,-0.141695629206859,
-0.850993704737257));
#9232=CARTESIAN_POINT('Ctrl Pts',(0.590422647829571,-0.181890537957859,
-0.830754510485543));
#9233=CARTESIAN_POINT('Ctrl Pts',(0.609616703125488,-0.201072148666545,
-0.816896541396381));
#9234=CARTESIAN_POINT('Ctrl Pts',(0.641117951819998,-0.223955109275652,
-0.792310597819928));
#9235=CARTESIAN_POINT('Ctrl Pts',(0.657208095763053,-0.232742381310829,
-0.779109323683612));
#9236=CARTESIAN_POINT('Ctrl Pts',(0.68964083160521,-0.244234834628584,-0.750552691816206));
#9237=CARTESIAN_POINT('Ctrl Pts',(0.705971972091755,-0.246942143572133,
-0.735185187071673));
#9238=CARTESIAN_POINT('Ctrl Pts',(0.735185187071673,-0.246942143572133,
-0.705971972091754));
#9239=CARTESIAN_POINT('Ctrl Pts',(0.750552691816206,-0.244234834628584,
-0.68964083160521));
#9240=CARTESIAN_POINT('Ctrl Pts',(0.779109323683612,-0.232742381310829,
-0.657208095763053));
#9241=CARTESIAN_POINT('Ctrl Pts',(0.792310597819928,-0.223955109275652,
-0.641117951819998));
#9242=CARTESIAN_POINT('Ctrl Pts',(0.816896541396381,-0.201072148666545,
-0.609616703125488));
#9243=CARTESIAN_POINT('Ctrl Pts',(0.830754510485543,-0.181890537957859,
-0.590422647829571));
#9244=CARTESIAN_POINT('Ctrl Pts',(0.850993704737257,-0.141695629206859,
-0.560922177770136));
#9245=CARTESIAN_POINT('Ctrl Pts',(0.85981294420286,-0.115492077056649,-0.54708917182331));
#9246=CARTESIAN_POINT('Ctrl Pts',(0.868149331745851,-0.0742967091364493,
-0.533674141594226));
#9247=CARTESIAN_POINT('Ctrl Pts',(0.870146645090731,-0.0609922781173484,
-0.530395067942936));
#9248=CARTESIAN_POINT('Ctrl Pts',(0.871530771444223,-0.0476300000000001,
-0.528110872004958));
#9249=CARTESIAN_POINT('',(0.989696097314,-0.04763,-0.242834539687906));
#9250=CARTESIAN_POINT('Origin',(0.,-0.04763,0.));
#9251=CARTESIAN_POINT('',(0.989696097314,-0.04763,0.242834539687906));
#9252=CARTESIAN_POINT('Ctrl Pts',(0.989696097314,-0.04763,-0.242834539687907));
#9253=CARTESIAN_POINT('Ctrl Pts',(0.990332542620729,-0.0609922781173483,
-0.24024064412003));
#9254=CARTESIAN_POINT('Ctrl Pts',(0.991238884025248,-0.0742967091364493,
-0.236509675094874));
#9255=CARTESIAN_POINT('Ctrl Pts',(0.994830026707808,-0.115492077056649,
-0.221129100087819));
#9256=CARTESIAN_POINT('Ctrl Pts',(0.998375294985966,-0.141695629206859,
-0.205111543747588));
#9257=CARTESIAN_POINT('Ctrl Pts',(1.00492400591205,-0.181890537957859,-0.169940289819232));
#9258=CARTESIAN_POINT('Ctrl Pts',(1.00869718865384,-0.201072148666545,-0.1465689792446));
#9259=CARTESIAN_POINT('Ctrl Pts',(1.01358704779679,-0.223955109275652,-0.106909345252087));
#9260=CARTESIAN_POINT('Ctrl Pts',(1.0156297872271,-0.232742381310829,-0.0861971848975942));
#9261=CARTESIAN_POINT('Ctrl Pts',(1.01837060663223,-0.244234834628584,-0.0430711894098823));
#9262=CARTESIAN_POINT('Ctrl Pts',(1.019052,-0.246942143572133,-0.0206568624125607));
#9263=CARTESIAN_POINT('Ctrl Pts',(1.019052,-0.246942143572133,0.0206568624125607));
#9264=CARTESIAN_POINT('Ctrl Pts',(1.01837060663223,-0.244234834628584,0.0430711894098823));
#9265=CARTESIAN_POINT('Ctrl Pts',(1.0156297872271,-0.232742381310829,0.0861971848975942));
#9266=CARTESIAN_POINT('Ctrl Pts',(1.01358704779679,-0.223955109275652,0.106909345252087));
#9267=CARTESIAN_POINT('Ctrl Pts',(1.00869718865384,-0.201072148666545,0.1465689792446));
#9268=CARTESIAN_POINT('Ctrl Pts',(1.00492400591205,-0.181890537957859,0.169940289819232));
#9269=CARTESIAN_POINT('Ctrl Pts',(0.998375294985966,-0.141695629206859,
0.205111543747588));
#9270=CARTESIAN_POINT('Ctrl Pts',(0.994830026707808,-0.115492077056649,
0.221129100087819));
#9271=CARTESIAN_POINT('Ctrl Pts',(0.991238884025248,-0.0742967091364492,
0.236509675094874));
#9272=CARTESIAN_POINT('Ctrl Pts',(0.990332542620729,-0.0609922781173483,
0.24024064412003));
#9273=CARTESIAN_POINT('Ctrl Pts',(0.989696097314,-0.04763,0.242834539687907));
#9274=CARTESIAN_POINT('Origin',(0.,-0.04763,0.));
#9275=CARTESIAN_POINT('Origin',(0.,-0.04763,0.));
#9276=CARTESIAN_POINT('',(0.238183666596899,-0.04763,0.951592097314));
#9277=CARTESIAN_POINT('Origin',(0.,-0.04763,0.));
#9278=CARTESIAN_POINT('Origin',(-1.94289029309402E-16,-0.04763,1.));
#9279=CARTESIAN_POINT('Origin',(-1.94289029309402E-16,0.,1.));
#9280=CARTESIAN_POINT('',(-0.2381836665969,-0.04763,0.951592097314));
#9281=CARTESIAN_POINT('Ctrl Pts',(-0.238183666596899,-0.0476299999999999,
0.951592097314));
#9282=CARTESIAN_POINT('Ctrl Pts',(-0.233157223576062,-0.0740444353928835,
0.952850216871763));
#9283=CARTESIAN_POINT('Ctrl Pts',(-0.223801617934946,-0.0999305678883309,
0.955173119738174));
#9284=CARTESIAN_POINT('Ctrl Pts',(-0.199966927975188,-0.142345102874864,
0.960411259488514));
#9285=CARTESIAN_POINT('Ctrl Pts',(-0.1868781821531,-0.159766064500479,0.963103647174702));
#9286=CARTESIAN_POINT('Ctrl Pts',(-0.15681442133453,-0.190326085855194,
0.968453058988463));
#9287=CARTESIAN_POINT('Ctrl Pts',(-0.139836317888043,-0.203463743702801,
0.971100730005489));
#9288=CARTESIAN_POINT('Ctrl Pts',(-0.104422493053067,-0.224161999508995,
0.975530745318961));
#9289=CARTESIAN_POINT('Ctrl Pts',(-0.0842175114474176,-0.232861760990032,
0.977553872336861));
#9290=CARTESIAN_POINT('Ctrl Pts',(-0.0421062857595701,-0.244251601209411,
0.980270995488453));
#9291=CARTESIAN_POINT('Ctrl Pts',(-0.0201990724523197,-0.246942143572133,
0.980948));
#9292=CARTESIAN_POINT('Ctrl Pts',(0.020199072452319,-0.246942143572133,
0.980948));
#9293=CARTESIAN_POINT('Ctrl Pts',(0.0421062857595694,-0.244251601209411,
0.980270995488454));
#9294=CARTESIAN_POINT('Ctrl Pts',(0.0842175114474169,-0.232861760990032,
0.977553872336861));
#9295=CARTESIAN_POINT('Ctrl Pts',(0.104422493053067,-0.224161999508995,
0.975530745318961));
#9296=CARTESIAN_POINT('Ctrl Pts',(0.139836317888042,-0.203463743702801,
0.971100730005489));
#9297=CARTESIAN_POINT('Ctrl Pts',(0.15681442133453,-0.190326085855194,0.968453058988463));
#9298=CARTESIAN_POINT('Ctrl Pts',(0.1868781821531,-0.15976606450048,0.963103647174702));
#9299=CARTESIAN_POINT('Ctrl Pts',(0.199966927975188,-0.142345102874864,
0.960411259488514));
#9300=CARTESIAN_POINT('Ctrl Pts',(0.223801617934945,-0.0999305678883309,
0.955173119738174));
#9301=CARTESIAN_POINT('Ctrl Pts',(0.233157223576061,-0.0740444353928835,
0.952850216871763));
#9302=CARTESIAN_POINT('Ctrl Pts',(0.238183666596899,-0.0476299999999999,
0.951592097314));
#9303=CARTESIAN_POINT('Origin',(-1.94289029309402E-16,-0.04763,1.));
#9304=CARTESIAN_POINT('Origin',(0.,-0.04763,0.));
#9305=CARTESIAN_POINT('',(-0.504455939115715,-0.04763,0.841298510752802));
#9306=CARTESIAN_POINT('Origin',(0.,-0.04763,0.));
#9307=CARTESIAN_POINT('Origin',(-0.707106781186548,-0.04763,0.707106781186547));
#9308=CARTESIAN_POINT('Origin',(-0.707106781186548,0.,0.707106781186547));
#9309=CARTESIAN_POINT('',(-0.841298510752802,-0.04763,0.504455939115715));
#9310=CARTESIAN_POINT('Ctrl Pts',(-0.841298510752802,-0.04763,0.504455939115715));
#9311=CARTESIAN_POINT('Ctrl Pts',(-0.838633903678357,-0.0740444353928835,
0.508899795931835));
#9312=CARTESIAN_POINT('Ctrl Pts',(-0.833661031856294,-0.0999305678883309,
0.517157748491652));
#9313=CARTESIAN_POINT('Ctrl Pts',(-0.820511285096538,-0.142345102874864,
0.537715343527944));
#9314=CARTESIAN_POINT('Ctrl Pts',(-0.813159949759,-0.159766064500479,0.548874290046456));
#9315=CARTESIAN_POINT('Ctrl Pts',(-0.795684265985089,-0.190326085855194,
0.573915184558107));
#9316=CARTESIAN_POINT('Ctrl Pts',(-0.78555112003688,-0.203463743702801,
0.587792702767295));
#9317=CARTESIAN_POINT('Ctrl Pts',(-0.763642258217233,-0.224161999508995,
0.615966552324775));
#9318=CARTESIAN_POINT('Ctrl Pts',(-0.750785745543687,-0.232861760990032,
0.631684198665438));
#9319=CARTESIAN_POINT('Ctrl Pts',(-0.722929908501543,-0.244251601209411,
0.663382628119203));
#9320=CARTESIAN_POINT('Ctrl Pts',(-0.707917883896095,-0.246942143572133,
0.679352081686668));
#9321=CARTESIAN_POINT('Ctrl Pts',(-0.679352081686668,-0.246942143572133,
0.707917883896095));
#9322=CARTESIAN_POINT('Ctrl Pts',(-0.663382628119203,-0.244251601209411,
0.722929908501544));
#9323=CARTESIAN_POINT('Ctrl Pts',(-0.631684198665438,-0.232861760990031,
0.750785745543687));
#9324=CARTESIAN_POINT('Ctrl Pts',(-0.615966552324775,-0.224161999508995,
0.763642258217233));
#9325=CARTESIAN_POINT('Ctrl Pts',(-0.587792702767295,-0.203463743702801,
0.78555112003688));
#9326=CARTESIAN_POINT('Ctrl Pts',(-0.573915184558107,-0.190326085855194,
0.795684265985088));
#9327=CARTESIAN_POINT('Ctrl Pts',(-0.548874290046456,-0.159766064500479,
0.813159949759));
#9328=CARTESIAN_POINT('Ctrl Pts',(-0.537715343527944,-0.142345102874864,
0.820511285096538));
#9329=CARTESIAN_POINT('Ctrl Pts',(-0.517157748491652,-0.0999305678883309,
0.833661031856294));
#9330=CARTESIAN_POINT('Ctrl Pts',(-0.508899795931835,-0.0740444353928835,
0.838633903678357));
#9331=CARTESIAN_POINT('Ctrl Pts',(-0.504455939115716,-0.04763,0.841298510752801));
#9332=CARTESIAN_POINT('Origin',(-0.707106781186548,-0.04763,0.707106781186547));
#9333=CARTESIAN_POINT('Origin',(0.,-0.04763,0.));
#9334=CARTESIAN_POINT('',(-0.951592097314,-0.04763,0.238183666596899));
#9335=CARTESIAN_POINT('Origin',(0.,-0.04763,0.));
#9336=CARTESIAN_POINT('Origin',(-1.,-0.04763,-1.11022302462516E-16));
#9337=CARTESIAN_POINT('Origin',(-1.,0.,-1.11022302462516E-16));
#9338=CARTESIAN_POINT('',(-0.951592097314,-0.04763,-0.2381836665969));
#9339=CARTESIAN_POINT('',(-0.980948,-0.246942143572133,1.08514323328844E-18));
#9340=CARTESIAN_POINT('Ctrl Pts',(-0.951592097314,-0.04763,-0.238183666596899));
#9341=CARTESIAN_POINT('Ctrl Pts',(-0.952850216871763,-0.0740444353928835,
-0.233157223576062));
#9342=CARTESIAN_POINT('Ctrl Pts',(-0.955173119738174,-0.0999305678883309,
-0.223801617934946));
#9343=CARTESIAN_POINT('Ctrl Pts',(-0.960411259488514,-0.142345102874864,
-0.199966927975188));
#9344=CARTESIAN_POINT('Ctrl Pts',(-0.963103647174702,-0.159766064500479,
-0.1868781821531));
#9345=CARTESIAN_POINT('Ctrl Pts',(-0.968453058988463,-0.190326085855194,
-0.15681442133453));
#9346=CARTESIAN_POINT('Ctrl Pts',(-0.971100730005489,-0.203463743702801,
-0.139836317888043));
#9347=CARTESIAN_POINT('Ctrl Pts',(-0.975530745318961,-0.224161999508995,
-0.104422493053067));
#9348=CARTESIAN_POINT('Ctrl Pts',(-0.977553872336861,-0.232861760990032,
-0.0842175114474175));
#9349=CARTESIAN_POINT('Ctrl Pts',(-0.980270995488453,-0.244251601209411,
-0.0421062857595699));
#9350=CARTESIAN_POINT('Ctrl Pts',(-0.980948,-0.246942143572133,-0.0201990724523195));
#9351=CARTESIAN_POINT('Ctrl Pts',(-0.980948,-0.246942143572133,-1.17961196366423E-16));
#9352=CARTESIAN_POINT('Origin',(-1.,-0.04763,-1.11022302462516E-16));
#9353=CARTESIAN_POINT('Ctrl Pts',(-0.980948,-0.246942143572133,-1.17961196366423E-16));
#9354=CARTESIAN_POINT('Ctrl Pts',(-0.980948,-0.246942143572133,0.0201990724523192));
#9355=CARTESIAN_POINT('Ctrl Pts',(-0.980270995488453,-0.244251601209411,
0.0421062857595695));
#9356=CARTESIAN_POINT('Ctrl Pts',(-0.977553872336861,-0.232861760990032,
0.0842175114474169));
#9357=CARTESIAN_POINT('Ctrl Pts',(-0.975530745318961,-0.224161999508995,
0.104422493053066));
#9358=CARTESIAN_POINT('Ctrl Pts',(-0.971100730005489,-0.203463743702801,
0.139836317888042));
#9359=CARTESIAN_POINT('Ctrl Pts',(-0.968453058988463,-0.190326085855194,
0.15681442133453));
#9360=CARTESIAN_POINT('Ctrl Pts',(-0.963103647174702,-0.15976606450048,
0.1868781821531));
#9361=CARTESIAN_POINT('Ctrl Pts',(-0.960411259488514,-0.142345102874864,
0.199966927975188));
#9362=CARTESIAN_POINT('Ctrl Pts',(-0.955173119738174,-0.099930567888331,
0.223801617934945));
#9363=CARTESIAN_POINT('Ctrl Pts',(-0.952850216871763,-0.0740444353928835,
0.233157223576061));
#9364=CARTESIAN_POINT('Ctrl Pts',(-0.951592097314,-0.04763,0.238183666596899));
#9365=CARTESIAN_POINT('Origin',(0.,-0.04763,0.));
#9366=CARTESIAN_POINT('',(-0.841298510752802,-0.04763,-0.504455939115715));
#9367=CARTESIAN_POINT('Origin',(0.,-0.04763,0.));
#9368=CARTESIAN_POINT('Origin',(-0.707106781186547,-0.04763,-0.707106781186548));
#9369=CARTESIAN_POINT('Origin',(-0.707106781186547,0.,-0.707106781186548));
#9370=CARTESIAN_POINT('',(-0.504455939115715,-0.04763,-0.841298510752802));
#9371=CARTESIAN_POINT('Ctrl Pts',(-0.504455939115715,-0.04763,-0.841298510752802));
#9372=CARTESIAN_POINT('Ctrl Pts',(-0.508899795931835,-0.0740444353928835,
-0.838633903678357));
#9373=CARTESIAN_POINT('Ctrl Pts',(-0.517157748491652,-0.0999305678883309,
-0.833661031856294));
#9374=CARTESIAN_POINT('Ctrl Pts',(-0.537715343527944,-0.142345102874864,
-0.820511285096538));
#9375=CARTESIAN_POINT('Ctrl Pts',(-0.548874290046456,-0.159766064500479,
-0.813159949759));
#9376=CARTESIAN_POINT('Ctrl Pts',(-0.573915184558107,-0.190326085855194,
-0.795684265985089));
#9377=CARTESIAN_POINT('Ctrl Pts',(-0.587792702767295,-0.203463743702801,
-0.78555112003688));
#9378=CARTESIAN_POINT('Ctrl Pts',(-0.615966552324775,-0.224161999508995,
-0.763642258217233));
#9379=CARTESIAN_POINT('Ctrl Pts',(-0.631684198665438,-0.232861760990032,
-0.750785745543687));
#9380=CARTESIAN_POINT('Ctrl Pts',(-0.663382628119203,-0.244251601209411,
-0.722929908501543));
#9381=CARTESIAN_POINT('Ctrl Pts',(-0.679352081686668,-0.246942143572133,
-0.707917883896095));
#9382=CARTESIAN_POINT('Ctrl Pts',(-0.707917883896095,-0.246942143572133,
-0.679352081686668));
#9383=CARTESIAN_POINT('Ctrl Pts',(-0.722929908501543,-0.244251601209411,
-0.663382628119203));
#9384=CARTESIAN_POINT('Ctrl Pts',(-0.750785745543687,-0.232861760990032,
-0.631684198665439));
#9385=CARTESIAN_POINT('Ctrl Pts',(-0.763642258217232,-0.224161999508995,
-0.615966552324775));
#9386=CARTESIAN_POINT('Ctrl Pts',(-0.78555112003688,-0.203463743702801,
-0.587792702767295));
#9387=CARTESIAN_POINT('Ctrl Pts',(-0.795684265985088,-0.190326085855194,
-0.573915184558107));
#9388=CARTESIAN_POINT('Ctrl Pts',(-0.813159949759,-0.15976606450048,-0.548874290046456));
#9389=CARTESIAN_POINT('Ctrl Pts',(-0.820511285096538,-0.142345102874864,
-0.537715343527944));
#9390=CARTESIAN_POINT('Ctrl Pts',(-0.833661031856294,-0.0999305678883311,
-0.517157748491652));
#9391=CARTESIAN_POINT('Ctrl Pts',(-0.838633903678357,-0.0740444353928836,
-0.508899795931835));
#9392=CARTESIAN_POINT('Ctrl Pts',(-0.841298510752801,-0.04763,-0.504455939115715));
#9393=CARTESIAN_POINT('Origin',(-0.707106781186547,-0.04763,-0.707106781186548));
#9394=CARTESIAN_POINT('Origin',(0.,-0.04763,0.));
#9395=CARTESIAN_POINT('',(-0.238183666596899,-0.04763,-0.951592097314));
#9396=CARTESIAN_POINT('Origin',(0.,-0.04763,0.));
#9397=CARTESIAN_POINT('Origin',(5.55111512312578E-17,-0.04763,-1.));
#9398=CARTESIAN_POINT('Origin',(5.55111512312578E-17,0.,-1.));
#9399=CARTESIAN_POINT('',(0.238183666596899,-0.04763,-0.951592097314));
#9400=CARTESIAN_POINT('Ctrl Pts',(0.238183666596899,-0.04763,-0.951592097314));
#9401=CARTESIAN_POINT('Ctrl Pts',(0.233157223576062,-0.0740444353928835,
-0.952850216871763));
#9402=CARTESIAN_POINT('Ctrl Pts',(0.223801617934946,-0.099930567888331,
-0.955173119738174));
#9403=CARTESIAN_POINT('Ctrl Pts',(0.199966927975188,-0.142345102874864,
-0.960411259488514));
#9404=CARTESIAN_POINT('Ctrl Pts',(0.1868781821531,-0.15976606450048,-0.963103647174702));
#9405=CARTESIAN_POINT('Ctrl Pts',(0.15681442133453,-0.190326085855194,-0.968453058988463));
#9406=CARTESIAN_POINT('Ctrl Pts',(0.139836317888042,-0.203463743702801,
-0.971100730005489));
#9407=CARTESIAN_POINT('Ctrl Pts',(0.104422493053067,-0.224161999508995,
-0.975530745318961));
#9408=CARTESIAN_POINT('Ctrl Pts',(0.0842175114474173,-0.232861760990032,
-0.977553872336861));
#9409=CARTESIAN_POINT('Ctrl Pts',(0.0421062857595698,-0.244251601209411,
-0.980270995488453));
#9410=CARTESIAN_POINT('Ctrl Pts',(0.0201990724523194,-0.246942143572133,
-0.980948));
#9411=CARTESIAN_POINT('Ctrl Pts',(-0.0201990724523193,-0.246942143572133,
-0.980948));
#9412=CARTESIAN_POINT('Ctrl Pts',(-0.0421062857595697,-0.244251601209411,
-0.980270995488453));
#9413=CARTESIAN_POINT('Ctrl Pts',(-0.0842175114474171,-0.232861760990032,
-0.977553872336861));
#9414=CARTESIAN_POINT('Ctrl Pts',(-0.104422493053067,-0.224161999508995,
-0.975530745318961));
#9415=CARTESIAN_POINT('Ctrl Pts',(-0.139836317888042,-0.203463743702801,
-0.971100730005489));
#9416=CARTESIAN_POINT('Ctrl Pts',(-0.15681442133453,-0.190326085855194,
-0.968453058988463));
#9417=CARTESIAN_POINT('Ctrl Pts',(-0.1868781821531,-0.15976606450048,-0.963103647174702));
#9418=CARTESIAN_POINT('Ctrl Pts',(-0.199966927975188,-0.142345102874864,
-0.960411259488514));
#9419=CARTESIAN_POINT('Ctrl Pts',(-0.223801617934945,-0.099930567888331,
-0.955173119738174));
#9420=CARTESIAN_POINT('Ctrl Pts',(-0.233157223576062,-0.0740444353928835,
-0.952850216871763));
#9421=CARTESIAN_POINT('Ctrl Pts',(-0.238183666596899,-0.0476299999999999,
-0.951592097314));
#9422=CARTESIAN_POINT('Origin',(5.55111512312578E-17,-0.04763,-1.));
#9423=CARTESIAN_POINT('Origin',(0.,-0.04763,0.));
#9424=CARTESIAN_POINT('',(0.504455939115715,-0.04763,-0.841298510752802));
#9425=CARTESIAN_POINT('Origin',(0.,-0.04763,0.));
#9426=CARTESIAN_POINT('Origin',(0.707106781186548,-0.04763,-0.707106781186547));
#9427=CARTESIAN_POINT('Origin',(0.707106781186548,0.,-0.707106781186547));
#9428=CARTESIAN_POINT('',(0.841298510752802,-0.04763,-0.504455939115715));
#9429=CARTESIAN_POINT('Ctrl Pts',(0.841298510752802,-0.04763,-0.504455939115715));
#9430=CARTESIAN_POINT('Ctrl Pts',(0.838633903678357,-0.0740444353928835,
-0.508899795931835));
#9431=CARTESIAN_POINT('Ctrl Pts',(0.833661031856294,-0.0999305678883309,
-0.517157748491652));
#9432=CARTESIAN_POINT('Ctrl Pts',(0.820511285096538,-0.142345102874864,
-0.537715343527944));
#9433=CARTESIAN_POINT('Ctrl Pts',(0.813159949759,-0.159766064500479,-0.548874290046456));
#9434=CARTESIAN_POINT('Ctrl Pts',(0.795684265985088,-0.190326085855194,
-0.573915184558107));
#9435=CARTESIAN_POINT('Ctrl Pts',(0.78555112003688,-0.203463743702801,-0.587792702767295));
#9436=CARTESIAN_POINT('Ctrl Pts',(0.763642258217233,-0.224161999508995,
-0.615966552324775));
#9437=CARTESIAN_POINT('Ctrl Pts',(0.750785745543687,-0.232861760990032,
-0.631684198665438));
#9438=CARTESIAN_POINT('Ctrl Pts',(0.722929908501543,-0.244251601209411,
-0.663382628119203));
#9439=CARTESIAN_POINT('Ctrl Pts',(0.707917883896095,-0.246942143572133,
-0.679352081686668));
#9440=CARTESIAN_POINT('Ctrl Pts',(0.679352081686668,-0.246942143572133,
-0.707917883896095));
#9441=CARTESIAN_POINT('Ctrl Pts',(0.663382628119203,-0.244251601209411,
-0.722929908501543));
#9442=CARTESIAN_POINT('Ctrl Pts',(0.631684198665438,-0.232861760990032,
-0.750785745543687));
#9443=CARTESIAN_POINT('Ctrl Pts',(0.615966552324775,-0.224161999508995,
-0.763642258217232));
#9444=CARTESIAN_POINT('Ctrl Pts',(0.587792702767295,-0.203463743702801,
-0.78555112003688));
#9445=CARTESIAN_POINT('Ctrl Pts',(0.573915184558107,-0.190326085855194,
-0.795684265985088));
#9446=CARTESIAN_POINT('Ctrl Pts',(0.548874290046456,-0.159766064500479,
-0.813159949759));
#9447=CARTESIAN_POINT('Ctrl Pts',(0.537715343527944,-0.142345102874864,
-0.820511285096538));
#9448=CARTESIAN_POINT('Ctrl Pts',(0.517157748491652,-0.099930567888331,
-0.833661031856294));
#9449=CARTESIAN_POINT('Ctrl Pts',(0.508899795931835,-0.0740444353928835,
-0.838633903678357));
#9450=CARTESIAN_POINT('Ctrl Pts',(0.504455939115715,-0.04763,-0.841298510752801));
#9451=CARTESIAN_POINT('Origin',(0.707106781186548,-0.04763,-0.707106781186547));
#9452=CARTESIAN_POINT('Origin',(0.,-0.166705,0.));
#9453=CARTESIAN_POINT('',(-0.980948,-0.28578,1.20131482833E-16));
#9454=CARTESIAN_POINT('Origin',(0.,-0.28578,0.));
#9455=CARTESIAN_POINT('',(-0.980948,-0.166705,1.20131482833E-16));
#9456=CARTESIAN_POINT('',(0.951592097314,-0.04763,0.238183666596899));
#9457=CARTESIAN_POINT('Origin',(0.,-0.04763,0.));
#9458=CARTESIAN_POINT('',(0.951592097314,-0.04763,-0.238183666596899));
#9459=CARTESIAN_POINT('Ctrl Pts',(0.951592097314,-0.04763,0.238183666596899));
#9460=CARTESIAN_POINT('Ctrl Pts',(0.952850216871763,-0.0740444353928835,
0.233157223576062));
#9461=CARTESIAN_POINT('Ctrl Pts',(0.955173119738174,-0.099930567888331,
0.223801617934945));
#9462=CARTESIAN_POINT('Ctrl Pts',(0.960411259488514,-0.142345102874864,
0.199966927975188));
#9463=CARTESIAN_POINT('Ctrl Pts',(0.963103647174702,-0.15976606450048,0.1868781821531));
#9464=CARTESIAN_POINT('Ctrl Pts',(0.968453058988463,-0.190326085855194,
0.15681442133453));
#9465=CARTESIAN_POINT('Ctrl Pts',(0.971100730005489,-0.203463743702801,
0.139836317888042));
#9466=CARTESIAN_POINT('Ctrl Pts',(0.975530745318961,-0.224161999508995,
0.104422493053067));
#9467=CARTESIAN_POINT('Ctrl Pts',(0.977553872336861,-0.232861760990032,
0.0842175114474172));
#9468=CARTESIAN_POINT('Ctrl Pts',(0.980270995488453,-0.244251601209411,
0.0421062857595697));
#9469=CARTESIAN_POINT('Ctrl Pts',(0.980948,-0.246942143572133,0.0201990724523194));
#9470=CARTESIAN_POINT('Ctrl Pts',(0.980948,-0.246942143572133,-0.0201990724523194));
#9471=CARTESIAN_POINT('Ctrl Pts',(0.980270995488453,-0.244251601209411,
-0.0421062857595697));
#9472=CARTESIAN_POINT('Ctrl Pts',(0.977553872336861,-0.232861760990032,
-0.0842175114474172));
#9473=CARTESIAN_POINT('Ctrl Pts',(0.975530745318961,-0.224161999508995,
-0.104422493053067));
#9474=CARTESIAN_POINT('Ctrl Pts',(0.971100730005489,-0.203463743702801,
-0.139836317888042));
#9475=CARTESIAN_POINT('Ctrl Pts',(0.968453058988463,-0.190326085855194,
-0.15681442133453));
#9476=CARTESIAN_POINT('Ctrl Pts',(0.963103647174702,-0.15976606450048,-0.1868781821531));
#9477=CARTESIAN_POINT('Ctrl Pts',(0.960411259488514,-0.142345102874864,
-0.199966927975188));
#9478=CARTESIAN_POINT('Ctrl Pts',(0.955173119738174,-0.099930567888331,
-0.223801617934945));
#9479=CARTESIAN_POINT('Ctrl Pts',(0.952850216871763,-0.0740444353928835,
-0.233157223576062));
#9480=CARTESIAN_POINT('Ctrl Pts',(0.951592097314,-0.0476299999999999,-0.238183666596899));
#9481=CARTESIAN_POINT('Origin',(0.,-0.04763,0.));
#9482=CARTESIAN_POINT('Origin',(0.,-0.04763,0.));
#9483=CARTESIAN_POINT('Origin',(1.,-0.04763,0.));
#9484=CARTESIAN_POINT('Origin',(1.,0.,0.));
#9485=CARTESIAN_POINT('Origin',(1.,-0.04763,0.));
#9486=CARTESIAN_POINT('Origin',(0.,-0.28578,0.));
#9487=CARTESIAN_POINT('Origin',(0.,-0.04763,0.));
#10583=UNCERTAINTY_MEASURE_WITH_UNIT(LENGTH_MEASURE(0.001),#10651,
'DISTANCE_ACCURACY_VALUE',
'Maximum model space distance between geometric entities at asserted c
onnectivities');
#10611=UNCERTAINTY_MEASURE_WITH_UNIT(LENGTH_MEASURE(0.001),#10651,
'DISTANCE_ACCURACY_VALUE',
'Maximum model space distance between geometric entities at asserted c
onnectivities');
#10622=(
GEOMETRIC_REPRESENTATION_CONTEXT(3)
GLOBAL_UNCERTAINTY_ASSIGNED_CONTEXT((#10583))
GLOBAL_UNIT_ASSIGNED_CONTEXT((#10651,#10653,#10654))
REPRESENTATION_CONTEXT('','3D')
);
#10650=(
GEOMETRIC_REPRESENTATION_CONTEXT(3)
GLOBAL_UNCERTAINTY_ASSIGNED_CONTEXT((#10611))
GLOBAL_UNIT_ASSIGNED_CONTEXT((#10651,#10653,#10654))
REPRESENTATION_CONTEXT('','3D')
);
#10651=(
LENGTH_UNIT()
NAMED_UNIT(*)
SI_UNIT(.CENTI.,.METRE.)
);
#10653=(
NAMED_UNIT(*)
PLANE_ANGLE_UNIT()
SI_UNIT($,.RADIAN.)
);
#10654=(
NAMED_UNIT(*)
SI_UNIT($,.STERADIAN.)
SOLID_ANGLE_UNIT()
);
#10665=SHAPE_DEFINITION_REPRESENTATION(#10703,#10804);
#10703=PRODUCT_DEFINITION_SHAPE('',$,#10843);
#10804=SHAPE_REPRESENTATION('',(#6141),#10622);
#10832=PRODUCT_DEFINITION_CONTEXT('part definition',#10948,'design');
#10843=PRODUCT_DEFINITION('Cage','Cage',#10881,#10832);
#10881=PRODUCT_DEFINITION_FORMATION('',$,#10960);
#10948=APPLICATION_CONTEXT(
'Core Data for Automotive Mechanical Design Process');
#10949=PRODUCT_CONTEXT('part definition',#10948,'mechanical');
#10960=PRODUCT('Cage','Cage','Cage',(#10949));
#11058=COLOUR_RGB('Grey',0.48,0.52,0.57);
#11059=FILL_AREA_STYLE_COLOUR('',#11058);
#11060=FILL_AREA_STYLE('',(#11059));
#11061=SURFACE_STYLE_FILL_AREA(#11060);
#11062=SURFACE_SIDE_STYLE('',(#11061));
#11063=SURFACE_STYLE_USAGE(.BOTH.,#11062);
#11064=PRESENTATION_STYLE_ASSIGNMENT((#11063));
ENDSEC;
END-ISO-10303-21;
